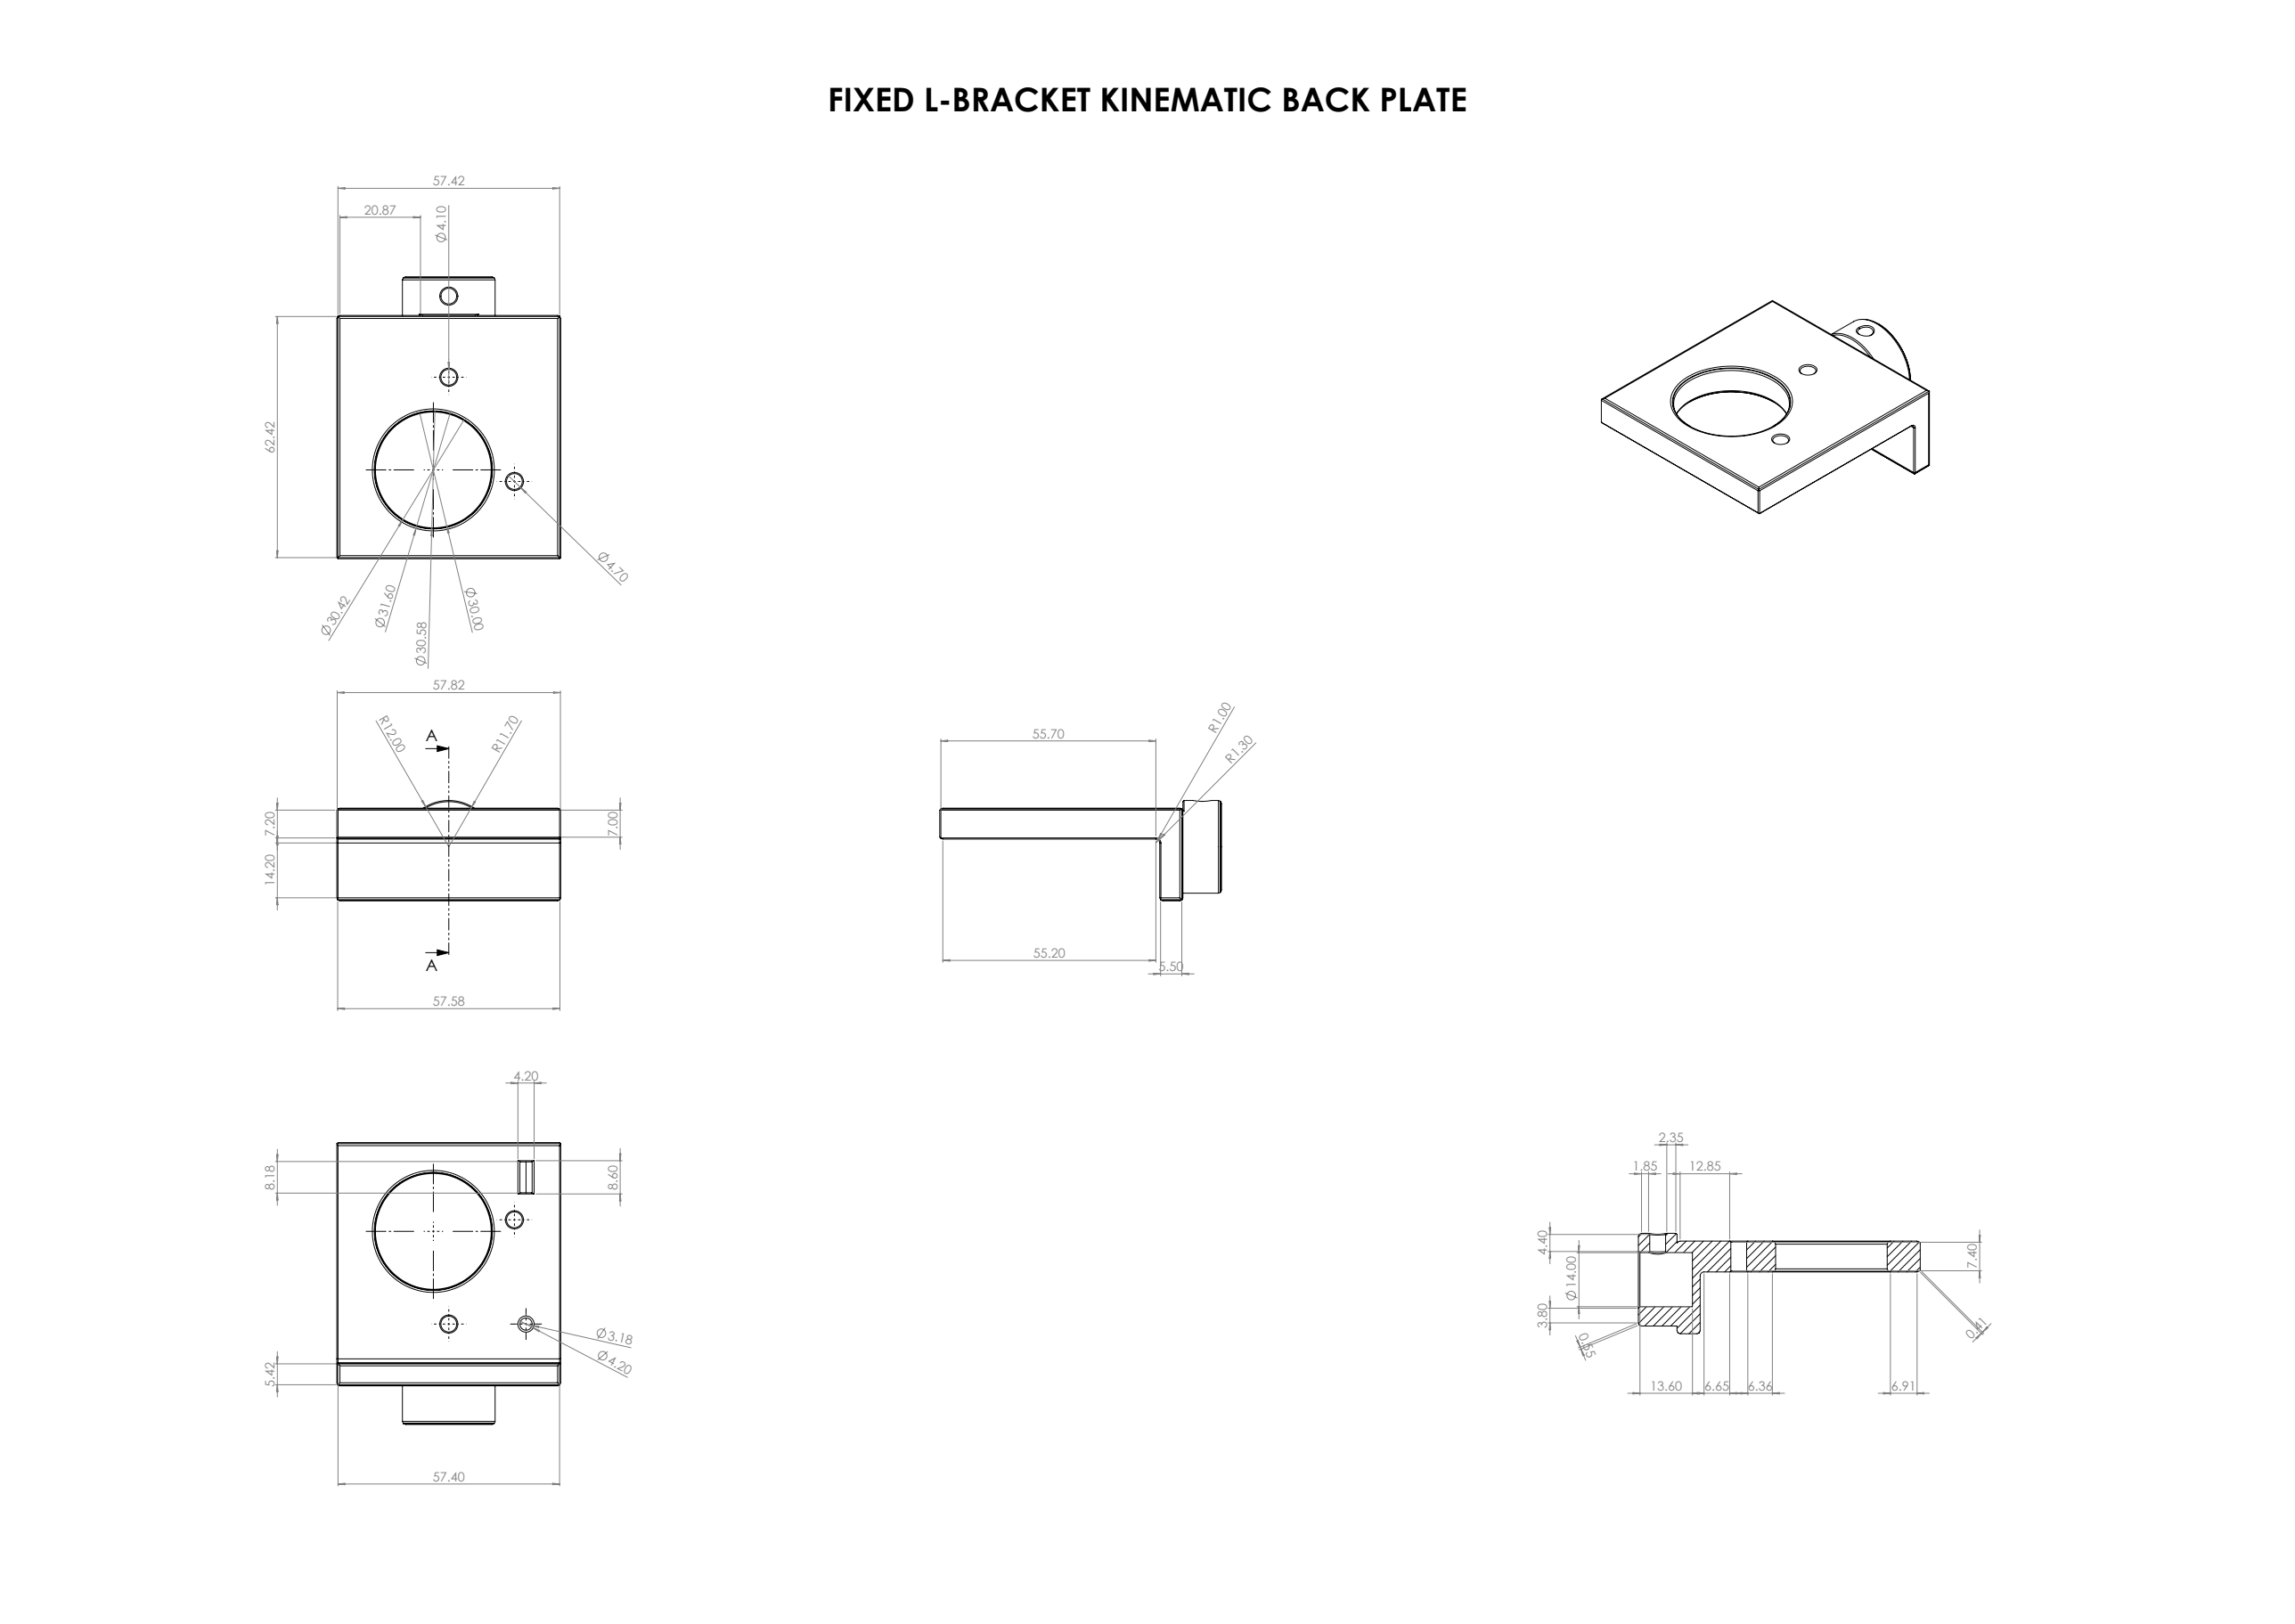
ISO-10303-21;
HEADER;
/* Generated by software containing ST-Developer
 * from STEP Tools, Inc. (www.steptools.com) 
 */

FILE_DESCRIPTION(
/* description */ (''),
/* implementation_level */ '2;1');

FILE_NAME(
/* name */ 
'04_Fixed_L-Bracket_Kinematic_Back_Plate.step',
/* time_stamp */ '2026-10-20T10:06:23-07:00',
/* author */ (''),
/* organization */ (''),
/* preprocessor_version */ 'ST-DEVELOPER v20.2',
/* originating_system */ 'Autodesk Translation Framework v15.15.0.0',
/* authorisation */ '');

FILE_SCHEMA (('AUTOMOTIVE_DESIGN { 1 0 10303 214 3 1 1 }'));
ENDSEC;

DATA;
#10=MECHANICAL_DESIGN_GEOMETRIC_PRESENTATION_REPRESENTATION('',(#468),#38611);
#96=ELLIPSE('',#16996,1.69705627484771,1.2);
#97=ELLIPSE('',#16998,1.69705627484771,1.2);
#130=(
BOUNDED_CURVE()
B_SPLINE_CURVE(2,(#27130,#27131,#27132),.UNSPECIFIED.,.F.,.F.)
B_SPLINE_CURVE_WITH_KNOTS((3,3),(0.245470547469808,0.342025381879347),
 .UNSPECIFIED.)
CURVE()
GEOMETRIC_REPRESENTATION_ITEM()
RATIONAL_B_SPLINE_CURVE((1.,1.,1.))
REPRESENTATION_ITEM('')
);
#131=(
BOUNDED_CURVE()
B_SPLINE_CURVE(2,(#27135,#27136,#27137),.UNSPECIFIED.,.F.,.F.)
B_SPLINE_CURVE_WITH_KNOTS((3,3),(0.165943124807515,0.262497959217054),
 .UNSPECIFIED.)
CURVE()
GEOMETRIC_REPRESENTATION_ITEM()
RATIONAL_B_SPLINE_CURVE((1.,1.,1.))
REPRESENTATION_ITEM('')
);
#440=SHAPE_REPRESENTATION_RELATIONSHIP('SRR','None',#38676,#454);
#454=ADVANCED_BREP_SHAPE_REPRESENTATION('',(#482),#38605);
#468=STYLED_ITEM('',(#38857),#482);
#482=MANIFOLD_SOLID_BREP('Bracket',#16242);
#501=B_SPLINE_SURFACE_WITH_KNOTS('',3,3,((#26897,#26898,#26899,#26900,#26901,
#26902,#26903,#26904,#26905,#26906,#26907,#26908,#26909,#26910,#26911,#26912,
#26913,#26914,#26915,#26916,#26917,#26918,#26919,#26920,#26921,#26922,#26923,
#26924,#26925,#26926),(#26927,#26928,#26929,#26930,#26931,#26932,#26933,
#26934,#26935,#26936,#26937,#26938,#26939,#26940,#26941,#26942,#26943,#26944,
#26945,#26946,#26947,#26948,#26949,#26950,#26951,#26952,#26953,#26954,#26955,
#26956),(#26957,#26958,#26959,#26960,#26961,#26962,#26963,#26964,#26965,
#26966,#26967,#26968,#26969,#26970,#26971,#26972,#26973,#26974,#26975,#26976,
#26977,#26978,#26979,#26980,#26981,#26982,#26983,#26984,#26985,#26986),
(#26987,#26988,#26989,#26990,#26991,#26992,#26993,#26994,#26995,#26996,
#26997,#26998,#26999,#27000,#27001,#27002,#27003,#27004,#27005,#27006,#27007,
#27008,#27009,#27010,#27011,#27012,#27013,#27014,#27015,#27016)),
 .UNSPECIFIED.,.F.,.T.,.F.,(4,4),(4,1,1,1,1,1,1,1,2,2,2,2,1,1,1,1,1,1,1,
2,2,4),(0.,1.),(0.,0.0483649312414982,0.0967298624829964,0.145094793724495,
0.193459724965993,0.241824656207491,0.290189587448989,0.326463285880113,
0.386919449931986,0.464302426118159,0.541687686804892,0.619072947491625,
0.677110750756395,0.735148554021165,0.793186357285935,0.851224160550705,
0.909261963815475,0.967299767080245,0.99631866871263,1.08337537360978,1.16076063429652,
1.23814589498325),.UNSPECIFIED.);
#502=B_SPLINE_SURFACE_WITH_KNOTS('',3,3,((#27146,#27147,#27148,#27149,#27150,
#27151,#27152,#27153,#27154,#27155,#27156,#27157,#27158,#27159,#27160,#27161,
#27162,#27163,#27164,#27165,#27166,#27167,#27168,#27169,#27170,#27171),
(#27172,#27173,#27174,#27175,#27176,#27177,#27178,#27179,#27180,#27181,
#27182,#27183,#27184,#27185,#27186,#27187,#27188,#27189,#27190,#27191,#27192,
#27193,#27194,#27195,#27196,#27197),(#27198,#27199,#27200,#27201,#27202,
#27203,#27204,#27205,#27206,#27207,#27208,#27209,#27210,#27211,#27212,#27213,
#27214,#27215,#27216,#27217,#27218,#27219,#27220,#27221,#27222,#27223),
(#27224,#27225,#27226,#27227,#27228,#27229,#27230,#27231,#27232,#27233,
#27234,#27235,#27236,#27237,#27238,#27239,#27240,#27241,#27242,#27243,#27244,
#27245,#27246,#27247,#27248,#27249)),.UNSPECIFIED.,.F.,.T.,.F.,(4,4),(4,
2,2,2,2,2,1,1,1,1,1,1,1,2,2,1,4),(0.,1.),(0.358934429201528,0.49197868985962,
0.564785636730508,0.596617469546802,0.699442998635822,0.77716819339067,
0.842568141080894,0.907968088771118,0.973368036461342,1.03876798415157,
1.07146795799668,1.10416793184179,1.16956787953201,1.30036777491246,1.39600843428647,
1.50005496459849,1.6041014949105),.UNSPECIFIED.);
#619=B_SPLINE_CURVE_WITH_KNOTS('',3,(#27021,#27022,#27023,#27024,#27025,
#27026,#27027,#27028,#27029,#27030,#27031,#27032,#27033,#27034,#27035,#27036,
#27037,#27038,#27039,#27040,#27041,#27042,#27043,#27044),.UNSPECIFIED.,
 .F.,.F.,(4,1,1,1,1,1,1,1,2,2,2,2,1,1,1,1,1,4),(0.,0.0483649312414982,0.0967298624829964,
0.145094793724495,0.193459724965993,0.241824656207491,0.290189587448989,
0.326463285880113,0.386919449931986,0.464302426118159,0.541687686804892,
0.619072947491625,0.677110750756395,0.735148554021165,0.793186357285935,
0.851224160550705,0.909261963815475,0.928609421237438),.UNSPECIFIED.);
#620=B_SPLINE_CURVE_WITH_KNOTS('',3,(#27045,#27046,#27047,#27048,#27049,
#27050,#27051,#27052,#27053,#27054),.UNSPECIFIED.,.F.,.F.,(4,1,1,2,2,4),
(0.928609421237438,0.967299767080245,0.99631866871263,1.08337537360978,
1.16076063429652,1.23814589498325),.UNSPECIFIED.);
#621=B_SPLINE_CURVE_WITH_KNOTS('',3,(#27055,#27056,#27057,#27058,#27059,
#27060,#27061,#27062,#27063,#27064,#27065,#27066,#27067,#27068,#27069,#27070,
#27071,#27072,#27073,#27074,#27075,#27076,#27077,#27078,#27079,#27080,#27081,
#27082,#27083,#27084),.UNSPECIFIED.,.T.,.F.,(4,2,2,1,1,1,1,1,1,1,2,2,2,
2,1,1,1,1,1,1,1,4),(-1.23814589498325,-1.16076063429652,-1.08337537360978,
-0.99631866871263,-0.967299767080245,-0.909261963815475,-0.851224160550705,
-0.793186357285935,-0.735148554021165,-0.677110750756395,-0.619072947491625,
-0.541687686804892,-0.464302426118159,-0.386919449931986,-0.326463285880113,
-0.290189587448989,-0.241824656207491,-0.193459724965993,-0.145094793724495,
-0.0967298624829964,-0.0483649312414982,0.),.UNSPECIFIED.);
#622=B_SPLINE_CURVE_WITH_KNOTS('',3,(#27097,#27098,#27099,#27100,#27101,
#27102,#27103,#27104,#27105,#27106,#27107,#27108,#27109,#27110,#27111,#27112),
 .UNSPECIFIED.,.F.,.F.,(4,2,2,2,2,2,1,1,4),(0.358934429201528,0.49197868985962,
0.564785636730508,0.596617469546802,0.699442998635822,0.77716819339067,
0.842568141080894,0.907968088771118,0.932576705821461),.UNSPECIFIED.);
#623=B_SPLINE_CURVE_WITH_KNOTS('',3,(#27113,#27114,#27115,#27116,#27117,
#27118,#27119,#27120,#27121,#27122,#27123,#27124,#27125,#27126),
 .UNSPECIFIED.,.F.,.F.,(4,1,1,1,1,1,2,2,1,4),(0.932576705821461,0.973368036461342,
1.03876798415157,1.07146795799668,1.10416793184179,1.16956787953201,1.30036777491246,
1.39600843428647,1.50005496459849,1.6041014949105),.UNSPECIFIED.);
#624=B_SPLINE_CURVE_WITH_KNOTS('',3,(#27253,#27254,#27255,#27256,#27257,
#27258,#27259,#27260,#27261,#27262),.UNSPECIFIED.,.F.,.F.,(4,1,2,2,1,4),
(-1.6041014949105,-1.50005496459849,-1.39600843428647,-1.30036777491246,
-1.16956787953201,-1.14109494863627),.UNSPECIFIED.);
#625=B_SPLINE_CURVE_WITH_KNOTS('',3,(#27264,#27265,#27266,#27267,#27268,
#27269,#27270,#27271,#27272,#27273,#27274,#27275),.UNSPECIFIED.,.F.,.F.,
(4,1,1,1,1,1,1,2,4),(-1.14109494863627,-1.10416793184179,-1.07146795799668,
-1.03876798415157,-0.973368036461342,-0.907968088771118,-0.842568141080894,
-0.77716819339067,-0.72405846300665),.UNSPECIFIED.);
#626=B_SPLINE_CURVE_WITH_KNOTS('',3,(#27276,#27277,#27278,#27279,#27280,
#27281,#27282,#27283,#27284,#27285,#27286,#27287),.UNSPECIFIED.,.F.,.F.,
(4,2,2,2,2,4),(-0.72405846300665,-0.699442998635822,-0.596617469546802,
-0.564785636730508,-0.49197868985962,-0.358934429201528),.UNSPECIFIED.);
#942=CYLINDRICAL_SURFACE('',#16994,1.2);
#943=CYLINDRICAL_SURFACE('',#16999,0.204999999999999);
#944=CYLINDRICAL_SURFACE('',#17006,0.7);
#945=CYLINDRICAL_SURFACE('',#17051,0.205);
#946=CYLINDRICAL_SURFACE('',#17055,0.205);
#947=CYLINDRICAL_SURFACE('',#17081,1.5);
#948=CYLINDRICAL_SURFACE('',#17097,0.1);
#1188=FACE_BOUND('',#3107,.T.);
#1189=FACE_BOUND('',#3114,.T.);
#1190=FACE_BOUND('',#3117,.T.);
#1191=FACE_BOUND('',#3146,.T.);
#1192=FACE_BOUND('',#3147,.T.);
#1193=FACE_BOUND('',#3148,.T.);
#1194=FACE_BOUND('',#3149,.T.);
#1195=FACE_BOUND('',#3150,.T.);
#1196=FACE_BOUND('',#3165,.T.);
#1197=FACE_BOUND('',#3166,.T.);
#1198=FACE_BOUND('',#3167,.T.);
#1410=CIRCLE('',#16992,1.2);
#1411=CIRCLE('',#16993,1.2);
#1412=CIRCLE('',#16995,1.2);
#1413=CIRCLE('',#16997,1.2);
#1414=CIRCLE('',#17001,1.17);
#1415=CIRCLE('',#17003,1.1787867965644);
#1416=CIRCLE('',#17005,1.1712132034356);
#1417=CIRCLE('',#17007,0.7);
#1418=CIRCLE('',#17008,0.7);
#1419=CIRCLE('',#17010,1.12);
#1420=CIRCLE('',#17012,0.74);
#1421=CIRCLE('',#17031,0.13);
#1422=CIRCLE('',#17042,0.21);
#1423=CIRCLE('',#17043,0.234999999999999);
#1424=CIRCLE('',#17044,1.58);
#1425=CIRCLE('',#17045,0.235);
#1426=CIRCLE('',#17047,0.158786796564404);
#1427=CIRCLE('',#17050,0.205);
#1428=CIRCLE('',#17052,0.205);
#1429=CIRCLE('',#17054,0.205);
#1430=CIRCLE('',#17056,0.205);
#1431=CIRCLE('',#17058,0.1);
#1432=CIRCLE('',#17061,0.1);
#1433=CIRCLE('',#17062,0.13);
#1434=CIRCLE('',#17065,1.5287867965644);
#1435=CIRCLE('',#17067,1.5212132034356);
#1436=CIRCLE('',#17069,0.235);
#1437=CIRCLE('',#17071,0.234999999999999);
#1438=CIRCLE('',#17072,1.58);
#1439=CIRCLE('',#17080,1.5);
#1440=CIRCLE('',#17082,1.5);
#1441=CIRCLE('',#17084,1.5287867965644);
#1442=CIRCLE('',#17086,1.5212132034356);
#1746=CONICAL_SURFACE('',#17000,1.185,0.785398163397445);
#1747=CONICAL_SURFACE('',#17002,1.1893933982822,0.392699081698718);
#1748=CONICAL_SURFACE('',#17004,1.175,0.785398163397451);
#1749=CONICAL_SURFACE('',#17009,1.1456066017178,1.17809724509618);
#1750=CONICAL_SURFACE('',#17046,0.184393398282202,1.17809724509617);
#1751=CONICAL_SURFACE('',#17048,0.115,0.785398163397448);
#1752=CONICAL_SURFACE('',#17049,0.22,0.785398163397453);
#1753=CONICAL_SURFACE('',#17053,0.22,0.785398163397438);
#1754=CONICAL_SURFACE('',#17057,0.115,0.785398163397456);
#1755=CONICAL_SURFACE('',#17060,0.115,0.785398163397456);
#1756=CONICAL_SURFACE('',#17064,1.5543933982822,1.17809724509617);
#1757=CONICAL_SURFACE('',#17066,1.525,0.785398163397449);
#1758=CONICAL_SURFACE('',#17068,0.22,0.785398163397452);
#1759=CONICAL_SURFACE('',#17073,0.22,0.785398163397437);
#1760=CONICAL_SURFACE('',#17079,1.5106066017178,0.392699081698724);
#1761=CONICAL_SURFACE('',#17083,1.5543933982822,1.17809724509617);
#1762=CONICAL_SURFACE('',#17085,1.525,0.785398163397448);
#1763=CONICAL_SURFACE('',#17087,1.5106066017178,0.392699081698721);
#1764=CONICAL_SURFACE('',#17090,0.72,0.785398163397448);
#2151=FACE_OUTER_BOUND('',#3097,.T.);
#2152=FACE_OUTER_BOUND('',#3098,.T.);
#2153=FACE_OUTER_BOUND('',#3099,.T.);
#2154=FACE_OUTER_BOUND('',#3100,.T.);
#2155=FACE_OUTER_BOUND('',#3101,.T.);
#2156=FACE_OUTER_BOUND('',#3102,.T.);
#2157=FACE_OUTER_BOUND('',#3103,.T.);
#2158=FACE_OUTER_BOUND('',#3104,.T.);
#2159=FACE_OUTER_BOUND('',#3105,.T.);
#2160=FACE_OUTER_BOUND('',#3106,.T.);
#2161=FACE_OUTER_BOUND('',#3108,.T.);
#2162=FACE_OUTER_BOUND('',#3109,.T.);
#2163=FACE_OUTER_BOUND('',#3110,.T.);
#2164=FACE_OUTER_BOUND('',#3111,.T.);
#2165=FACE_OUTER_BOUND('',#3112,.T.);
#2166=FACE_OUTER_BOUND('',#3113,.T.);
#2167=FACE_OUTER_BOUND('',#3115,.T.);
#2168=FACE_OUTER_BOUND('',#3116,.T.);
#2169=FACE_OUTER_BOUND('',#3118,.T.);
#2170=FACE_OUTER_BOUND('',#3119,.T.);
#2171=FACE_OUTER_BOUND('',#3120,.T.);
#2172=FACE_OUTER_BOUND('',#3121,.T.);
#2173=FACE_OUTER_BOUND('',#3122,.T.);
#2174=FACE_OUTER_BOUND('',#3123,.T.);
#2175=FACE_OUTER_BOUND('',#3124,.T.);
#2176=FACE_OUTER_BOUND('',#3125,.T.);
#2177=FACE_OUTER_BOUND('',#3126,.T.);
#2178=FACE_OUTER_BOUND('',#3127,.T.);
#2179=FACE_OUTER_BOUND('',#3128,.T.);
#2180=FACE_OUTER_BOUND('',#3129,.T.);
#2181=FACE_OUTER_BOUND('',#3130,.T.);
#2182=FACE_OUTER_BOUND('',#3131,.T.);
#2183=FACE_OUTER_BOUND('',#3132,.T.);
#2184=FACE_OUTER_BOUND('',#3133,.T.);
#2185=FACE_OUTER_BOUND('',#3134,.T.);
#2186=FACE_OUTER_BOUND('',#3135,.T.);
#2187=FACE_OUTER_BOUND('',#3136,.T.);
#2188=FACE_OUTER_BOUND('',#3137,.T.);
#2189=FACE_OUTER_BOUND('',#3138,.T.);
#2190=FACE_OUTER_BOUND('',#3139,.T.);
#2191=FACE_OUTER_BOUND('',#3140,.T.);
#2192=FACE_OUTER_BOUND('',#3141,.T.);
#2193=FACE_OUTER_BOUND('',#3142,.T.);
#2194=FACE_OUTER_BOUND('',#3143,.T.);
#2195=FACE_OUTER_BOUND('',#3144,.T.);
#2196=FACE_OUTER_BOUND('',#3145,.T.);
#2197=FACE_OUTER_BOUND('',#3151,.T.);
#2198=FACE_OUTER_BOUND('',#3152,.T.);
#2199=FACE_OUTER_BOUND('',#3153,.T.);
#2200=FACE_OUTER_BOUND('',#3154,.T.);
#2201=FACE_OUTER_BOUND('',#3155,.T.);
#2202=FACE_OUTER_BOUND('',#3156,.T.);
#2203=FACE_OUTER_BOUND('',#3157,.T.);
#2204=FACE_OUTER_BOUND('',#3158,.T.);
#2205=FACE_OUTER_BOUND('',#3159,.T.);
#2206=FACE_OUTER_BOUND('',#3160,.T.);
#2207=FACE_OUTER_BOUND('',#3161,.T.);
#2208=FACE_OUTER_BOUND('',#3162,.T.);
#2209=FACE_OUTER_BOUND('',#3163,.T.);
#2210=FACE_OUTER_BOUND('',#3164,.T.);
#2211=FACE_OUTER_BOUND('',#3168,.T.);
#2212=FACE_OUTER_BOUND('',#3169,.T.);
#2213=FACE_OUTER_BOUND('',#3170,.T.);
#2214=FACE_OUTER_BOUND('',#3171,.T.);
#2215=FACE_OUTER_BOUND('',#3172,.T.);
#2216=FACE_OUTER_BOUND('',#3173,.T.);
#2217=FACE_OUTER_BOUND('',#3174,.T.);
#2218=FACE_OUTER_BOUND('',#3175,.T.);
#2219=FACE_OUTER_BOUND('',#3176,.T.);
#2220=FACE_OUTER_BOUND('',#3177,.T.);
#2221=FACE_OUTER_BOUND('',#3178,.T.);
#2222=FACE_OUTER_BOUND('',#3179,.T.);
#2223=FACE_OUTER_BOUND('',#3180,.T.);
#2224=FACE_OUTER_BOUND('',#3181,.T.);
#2225=FACE_OUTER_BOUND('',#3182,.T.);
#2226=FACE_OUTER_BOUND('',#3183,.T.);
#2227=FACE_OUTER_BOUND('',#3184,.T.);
#2228=FACE_OUTER_BOUND('',#3185,.T.);
#2229=FACE_OUTER_BOUND('',#3186,.T.);
#2230=FACE_OUTER_BOUND('',#3187,.T.);
#2231=FACE_OUTER_BOUND('',#3188,.T.);
#3097=EDGE_LOOP('',(#11825,#11826,#11827,#11828,#11829,#11830));
#3098=EDGE_LOOP('',(#11831,#11832,#11833,#11834,#11835));
#3099=EDGE_LOOP('',(#11836,#11837,#11838,#11839,#11840));
#3100=EDGE_LOOP('',(#11841,#11842,#11843,#11844));
#3101=EDGE_LOOP('',(#11845,#11846,#11847,#11848));
#3102=EDGE_LOOP('',(#11849,#11850,#11851,#11852));
#3103=EDGE_LOOP('',(#11853,#11854,#11855,#11856));
#3104=EDGE_LOOP('',(#11857,#11858,#11859,#11860,#11861,#11862,#11863));
#3105=EDGE_LOOP('',(#11864,#11865,#11866,#11867,#11868));
#3106=EDGE_LOOP('',(#11869,#11870,#11871,#11872,#11873,#11874,#11875,#11876));
#3107=EDGE_LOOP('',(#11877));
#3108=EDGE_LOOP('',(#11878,#11879,#11880,#11881,#11882,#11883));
#3109=EDGE_LOOP('',(#11884,#11885,#11886,#11887));
#3110=EDGE_LOOP('',(#11888,#11889,#11890,#11891));
#3111=EDGE_LOOP('',(#11892,#11893,#11894,#11895));
#3112=EDGE_LOOP('',(#11896,#11897,#11898,#11899,#11900,#11901,#11902));
#3113=EDGE_LOOP('',(#11903,#11904,#11905,#11906));
#3114=EDGE_LOOP('',(#11907,#11908,#11909));
#3115=EDGE_LOOP('',(#11910,#11911,#11912,#11913));
#3116=EDGE_LOOP('',(#11914));
#3117=EDGE_LOOP('',(#11915));
#3118=EDGE_LOOP('',(#11916,#11917,#11918,#11919));
#3119=EDGE_LOOP('',(#11920,#11921,#11922,#11923));
#3120=EDGE_LOOP('',(#11924,#11925,#11926,#11927));
#3121=EDGE_LOOP('',(#11928,#11929,#11930,#11931));
#3122=EDGE_LOOP('',(#11932,#11933,#11934,#11935,#11936));
#3123=EDGE_LOOP('',(#11937,#11938,#11939,#11940));
#3124=EDGE_LOOP('',(#11941,#11942,#11943,#11944,#11945,#11946));
#3125=EDGE_LOOP('',(#11947,#11948,#11949,#11950,#11951,#11952));
#3126=EDGE_LOOP('',(#11953,#11954,#11955,#11956,#11957,#11958));
#3127=EDGE_LOOP('',(#11959,#11960,#11961,#11962));
#3128=EDGE_LOOP('',(#11963,#11964,#11965,#11966));
#3129=EDGE_LOOP('',(#11967,#11968,#11969,#11970,#11971,#11972,#11973));
#3130=EDGE_LOOP('',(#11974,#11975,#11976,#11977,#11978,#11979));
#3131=EDGE_LOOP('',(#11980,#11981,#11982,#11983,#11984));
#3132=EDGE_LOOP('',(#11985,#11986,#11987,#11988));
#3133=EDGE_LOOP('',(#11989,#11990,#11991,#11992,#11993));
#3134=EDGE_LOOP('',(#11994,#11995,#11996,#11997,#11998,#11999,#12000));
#3135=EDGE_LOOP('',(#12001,#12002,#12003,#12004,#12005,#12006,#12007));
#3136=EDGE_LOOP('',(#12008,#12009,#12010,#12011,#12012));
#3137=EDGE_LOOP('',(#12013,#12014,#12015,#12016,#12017,#12018));
#3138=EDGE_LOOP('',(#12019,#12020,#12021,#12022,#12023,#12024));
#3139=EDGE_LOOP('',(#12025,#12026,#12027,#12028));
#3140=EDGE_LOOP('',(#12029,#12030,#12031,#12032));
#3141=EDGE_LOOP('',(#12033,#12034,#12035,#12036,#12037,#12038));
#3142=EDGE_LOOP('',(#12039,#12040,#12041,#12042,#12043,#12044));
#3143=EDGE_LOOP('',(#12045,#12046,#12047));
#3144=EDGE_LOOP('',(#12048,#12049,#12050,#12051,#12052,#12053));
#3145=EDGE_LOOP('',(#12054,#12055,#12056,#12057));
#3146=EDGE_LOOP('',(#12058));
#3147=EDGE_LOOP('',(#12059));
#3148=EDGE_LOOP('',(#12060));
#3149=EDGE_LOOP('',(#12061));
#3150=EDGE_LOOP('',(#12062,#12063,#12064,#12065));
#3151=EDGE_LOOP('',(#12066,#12067,#12068,#12069));
#3152=EDGE_LOOP('',(#12070,#12071,#12072));
#3153=EDGE_LOOP('',(#12073,#12074,#12075,#12076));
#3154=EDGE_LOOP('',(#12077,#12078,#12079,#12080));
#3155=EDGE_LOOP('',(#12081,#12082,#12083,#12084));
#3156=EDGE_LOOP('',(#12085,#12086,#12087,#12088));
#3157=EDGE_LOOP('',(#12089,#12090,#12091,#12092));
#3158=EDGE_LOOP('',(#12093,#12094,#12095,#12096));
#3159=EDGE_LOOP('',(#12097,#12098,#12099,#12100));
#3160=EDGE_LOOP('',(#12101,#12102,#12103,#12104,#12105,#12106,#12107));
#3161=EDGE_LOOP('',(#12108,#12109,#12110,#12111));
#3162=EDGE_LOOP('',(#12112,#12113,#12114,#12115));
#3163=EDGE_LOOP('',(#12116,#12117,#12118,#12119));
#3164=EDGE_LOOP('',(#12120,#12121,#12122,#12123));
#3165=EDGE_LOOP('',(#12124));
#3166=EDGE_LOOP('',(#12125));
#3167=EDGE_LOOP('',(#12126));
#3168=EDGE_LOOP('',(#12127,#12128,#12129,#12130));
#3169=EDGE_LOOP('',(#12131,#12132,#12133,#12134));
#3170=EDGE_LOOP('',(#12135,#12136,#12137,#12138));
#3171=EDGE_LOOP('',(#12139,#12140,#12141,#12142));
#3172=EDGE_LOOP('',(#12143,#12144,#12145,#12146));
#3173=EDGE_LOOP('',(#12147,#12148,#12149,#12150,#12151,#12152,#12153,#12154,
#12155,#12156,#12157,#12158,#12159,#12160));
#3174=EDGE_LOOP('',(#12161,#12162,#12163,#12164));
#3175=EDGE_LOOP('',(#12165,#12166,#12167,#12168));
#3176=EDGE_LOOP('',(#12169,#12170,#12171,#12172));
#3177=EDGE_LOOP('',(#12173,#12174,#12175,#12176));
#3178=EDGE_LOOP('',(#12177,#12178,#12179,#12180));
#3179=EDGE_LOOP('',(#12181,#12182,#12183,#12184,#12185,#12186));
#3180=EDGE_LOOP('',(#12187,#12188,#12189));
#3181=EDGE_LOOP('',(#12190,#12191,#12192,#12193));
#3182=EDGE_LOOP('',(#12194));
#3183=EDGE_LOOP('',(#12195,#12196));
#3184=EDGE_LOOP('',(#12197,#12198,#12199,#12200,#12201,#12202));
#3185=EDGE_LOOP('',(#12203,#12204,#12205,#12206,#12207,#12208));
#3186=EDGE_LOOP('',(#12209,#12210,#12211,#12212,#12213,#12214));
#3187=EDGE_LOOP('',(#12215,#12216,#12217,#12218));
#3188=EDGE_LOOP('',(#12219,#12220,#12221,#12222));
#4211=LINE('',#26838,#5435);
#4212=LINE('',#26840,#5436);
#4213=LINE('',#26842,#5437);
#4214=LINE('',#26844,#5438);
#4215=LINE('',#26846,#5439);
#4216=LINE('',#26847,#5440);
#4217=LINE('',#26850,#5441);
#4218=LINE('',#26852,#5442);
#4219=LINE('',#26854,#5443);
#4220=LINE('',#26855,#5444);
#4221=LINE('',#26858,#5445);
#4222=LINE('',#26860,#5446);
#4223=LINE('',#26861,#5447);
#4224=LINE('',#26864,#5448);
#4225=LINE('',#26866,#5449);
#4226=LINE('',#26867,#5450);
#4227=LINE('',#26871,#5451);
#4228=LINE('',#26873,#5452);
#4229=LINE('',#26875,#5453);
#4230=LINE('',#26876,#5454);
#4231=LINE('',#26879,#5455);
#4232=LINE('',#26881,#5456);
#4233=LINE('',#26882,#5457);
#4234=LINE('',#26885,#5458);
#4235=LINE('',#26887,#5459);
#4236=LINE('',#26888,#5460);
#4237=LINE('',#26891,#5461);
#4238=LINE('',#26896,#5462);
#4239=LINE('',#27019,#5463);
#4240=LINE('',#27088,#5464);
#4241=LINE('',#27127,#5465);
#4242=LINE('',#27141,#5466);
#4243=LINE('',#27145,#5467);
#4244=LINE('',#27251,#5468);
#4245=LINE('',#27292,#5469);
#4246=LINE('',#27296,#5470);
#4247=LINE('',#27304,#5471);
#4248=LINE('',#27306,#5472);
#4249=LINE('',#27308,#5473);
#4250=LINE('',#27309,#5474);
#4251=LINE('',#27313,#5475);
#4252=LINE('',#27314,#5476);
#4253=LINE('',#27315,#5477);
#4254=LINE('',#27317,#5478);
#4255=LINE('',#27318,#5479);
#4256=LINE('',#27320,#5480);
#4257=LINE('',#27321,#5481);
#4258=LINE('',#27324,#5482);
#4259=LINE('',#27326,#5483);
#4260=LINE('',#27327,#5484);
#4261=LINE('',#27332,#5485);
#4262=LINE('',#27334,#5486);
#4263=LINE('',#27336,#5487);
#4264=LINE('',#27338,#5488);
#4265=LINE('',#27340,#5489);
#4266=LINE('',#27341,#5490);
#4267=LINE('',#27344,#5491);
#4268=LINE('',#27346,#5492);
#4269=LINE('',#27348,#5493);
#4270=LINE('',#27350,#5494);
#4271=LINE('',#27351,#5495);
#4272=LINE('',#27354,#5496);
#4273=LINE('',#27356,#5497);
#4274=LINE('',#27358,#5498);
#4275=LINE('',#27359,#5499);
#4276=LINE('',#27362,#5500);
#4277=LINE('',#27363,#5501);
#4278=LINE('',#27366,#5502);
#4279=LINE('',#27368,#5503);
#4280=LINE('',#27369,#5504);
#4281=LINE('',#27371,#5505);
#4282=LINE('',#27373,#5506);
#4283=LINE('',#27375,#5507);
#4284=LINE('',#27377,#5508);
#4285=LINE('',#27378,#5509);
#4286=LINE('',#27380,#5510);
#4287=LINE('',#27382,#5511);
#4288=LINE('',#27383,#5512);
#4289=LINE('',#27385,#5513);
#4290=LINE('',#27389,#5514);
#4291=LINE('',#27391,#5515);
#4292=LINE('',#27392,#5516);
#4293=LINE('',#27393,#5517);
#4294=LINE('',#27396,#5518);
#4295=LINE('',#27397,#5519);
#4296=LINE('',#27400,#5520);
#4297=LINE('',#27402,#5521);
#4298=LINE('',#27404,#5522);
#4299=LINE('',#27406,#5523);
#4300=LINE('',#27408,#5524);
#4301=LINE('',#27409,#5525);
#4302=LINE('',#27412,#5526);
#4303=LINE('',#27416,#5527);
#4304=LINE('',#27417,#5528);
#4305=LINE('',#27420,#5529);
#4306=LINE('',#27421,#5530);
#4307=LINE('',#27423,#5531);
#4308=LINE('',#27424,#5532);
#4309=LINE('',#27427,#5533);
#4310=LINE('',#27429,#5534);
#4311=LINE('',#27430,#5535);
#4312=LINE('',#27434,#5536);
#4313=LINE('',#27436,#5537);
#4314=LINE('',#27438,#5538);
#4315=LINE('',#27439,#5539);
#4316=LINE('',#27443,#5540);
#4317=LINE('',#27445,#5541);
#4318=LINE('',#27447,#5542);
#4319=LINE('',#27448,#5543);
#4320=LINE('',#27452,#5544);
#4321=LINE('',#27453,#5545);
#4322=LINE('',#27454,#5546);
#4323=LINE('',#27455,#5547);
#4324=LINE('',#27457,#5548);
#4325=LINE('',#27459,#5549);
#4326=LINE('',#27461,#5550);
#4327=LINE('',#27462,#5551);
#4328=LINE('',#27465,#5552);
#4329=LINE('',#27466,#5553);
#4330=LINE('',#27469,#5554);
#4331=LINE('',#27470,#5555);
#4332=LINE('',#27472,#5556);
#4333=LINE('',#27473,#5557);
#4334=LINE('',#27484,#5558);
#4335=LINE('',#27488,#5559);
#4336=LINE('',#27491,#5560);
#4337=LINE('',#27495,#5561);
#4338=LINE('',#27499,#5562);
#4339=LINE('',#27503,#5563);
#4340=LINE('',#27515,#5564);
#4341=LINE('',#27518,#5565);
#4342=LINE('',#27523,#5566);
#4343=LINE('',#27527,#5567);
#4344=LINE('',#27529,#5568);
#4345=LINE('',#27531,#5569);
#4346=LINE('',#27532,#5570);
#4347=LINE('',#27538,#5571);
#4348=LINE('',#27540,#5572);
#4349=LINE('',#27541,#5573);
#4350=LINE('',#27542,#5574);
#4351=LINE('',#27544,#5575);
#4352=LINE('',#27545,#5576);
#4353=LINE('',#27546,#5577);
#4354=LINE('',#27550,#5578);
#4355=LINE('',#27551,#5579);
#4356=LINE('',#27554,#5580);
#4357=LINE('',#27559,#5581);
#4358=LINE('',#27563,#5582);
#4359=LINE('',#27566,#5583);
#4360=LINE('',#27569,#5584);
#4361=LINE('',#27571,#5585);
#4362=LINE('',#27574,#5586);
#4363=LINE('',#27578,#5587);
#4364=LINE('',#27582,#5588);
#5435=VECTOR('',#19526,1.);
#5436=VECTOR('',#19527,1.);
#5437=VECTOR('',#19528,1.);
#5438=VECTOR('',#19529,1.);
#5439=VECTOR('',#19530,1.);
#5440=VECTOR('',#19531,1.);
#5441=VECTOR('',#19534,1.);
#5442=VECTOR('',#19535,1.);
#5443=VECTOR('',#19536,1.);
#5444=VECTOR('',#19537,1.);
#5445=VECTOR('',#19540,1.);
#5446=VECTOR('',#19541,1.);
#5447=VECTOR('',#19542,1.);
#5448=VECTOR('',#19545,1.);
#5449=VECTOR('',#19546,1.);
#5450=VECTOR('',#19547,1.);
#5451=VECTOR('',#19550,1.);
#5452=VECTOR('',#19551,1.);
#5453=VECTOR('',#19552,1.);
#5454=VECTOR('',#19553,1.);
#5455=VECTOR('',#19556,1.);
#5456=VECTOR('',#19557,1.);
#5457=VECTOR('',#19558,1.);
#5458=VECTOR('',#19561,1.);
#5459=VECTOR('',#19562,1.);
#5460=VECTOR('',#19563,1.);
#5461=VECTOR('',#19566,1.);
#5462=VECTOR('',#19571,1.);
#5463=VECTOR('',#19572,1.);
#5464=VECTOR('',#19577,1.2);
#5465=VECTOR('',#19586,0.204999999999999);
#5466=VECTOR('',#19595,1.1893933982822);
#5467=VECTOR('',#19600,1.175);
#5468=VECTOR('',#19601,1.);
#5469=VECTOR('',#19606,0.7);
#5470=VECTOR('',#19611,1.1456066017178);
#5471=VECTOR('',#19620,1.);
#5472=VECTOR('',#19621,1.);
#5473=VECTOR('',#19622,1.);
#5474=VECTOR('',#19623,1.);
#5475=VECTOR('',#19626,1.);
#5476=VECTOR('',#19627,1.);
#5477=VECTOR('',#19628,1.);
#5478=VECTOR('',#19631,1.);
#5479=VECTOR('',#19632,1.);
#5480=VECTOR('',#19635,1.);
#5481=VECTOR('',#19636,1.);
#5482=VECTOR('',#19639,1.);
#5483=VECTOR('',#19640,1.);
#5484=VECTOR('',#19641,1.);
#5485=VECTOR('',#19646,1.);
#5486=VECTOR('',#19647,1.);
#5487=VECTOR('',#19648,1.);
#5488=VECTOR('',#19649,1.);
#5489=VECTOR('',#19650,1.);
#5490=VECTOR('',#19651,1.);
#5491=VECTOR('',#19654,1.);
#5492=VECTOR('',#19655,1.);
#5493=VECTOR('',#19656,1.);
#5494=VECTOR('',#19657,1.);
#5495=VECTOR('',#19658,1.);
#5496=VECTOR('',#19661,1.);
#5497=VECTOR('',#19662,1.);
#5498=VECTOR('',#19663,1.);
#5499=VECTOR('',#19664,1.);
#5500=VECTOR('',#19667,1.);
#5501=VECTOR('',#19668,1.);
#5502=VECTOR('',#19671,1.);
#5503=VECTOR('',#19672,1.);
#5504=VECTOR('',#19673,1.);
#5505=VECTOR('',#19676,1.);
#5506=VECTOR('',#19677,1.);
#5507=VECTOR('',#19678,1.);
#5508=VECTOR('',#19679,1.);
#5509=VECTOR('',#19680,1.);
#5510=VECTOR('',#19683,1.);
#5511=VECTOR('',#19684,1.);
#5512=VECTOR('',#19685,1.);
#5513=VECTOR('',#19688,1.);
#5514=VECTOR('',#19691,1.);
#5515=VECTOR('',#19692,1.);
#5516=VECTOR('',#19693,1.);
#5517=VECTOR('',#19694,1.);
#5518=VECTOR('',#19697,1.);
#5519=VECTOR('',#19698,1.);
#5520=VECTOR('',#19701,1.);
#5521=VECTOR('',#19702,1.);
#5522=VECTOR('',#19703,1.);
#5523=VECTOR('',#19704,1.);
#5524=VECTOR('',#19705,1.);
#5525=VECTOR('',#19706,1.);
#5526=VECTOR('',#19709,1.);
#5527=VECTOR('',#19712,1.);
#5528=VECTOR('',#19713,1.);
#5529=VECTOR('',#19716,1.);
#5530=VECTOR('',#19717,1.);
#5531=VECTOR('',#19720,1.);
#5532=VECTOR('',#19721,1.);
#5533=VECTOR('',#19724,1.);
#5534=VECTOR('',#19725,1.);
#5535=VECTOR('',#19726,1.);
#5536=VECTOR('',#19729,1.);
#5537=VECTOR('',#19730,1.);
#5538=VECTOR('',#19731,1.);
#5539=VECTOR('',#19732,1.);
#5540=VECTOR('',#19735,1.);
#5541=VECTOR('',#19736,1.);
#5542=VECTOR('',#19737,1.);
#5543=VECTOR('',#19738,1.);
#5544=VECTOR('',#19741,1.);
#5545=VECTOR('',#19742,1.);
#5546=VECTOR('',#19743,1.);
#5547=VECTOR('',#19744,1.);
#5548=VECTOR('',#19747,1.);
#5549=VECTOR('',#19748,1.);
#5550=VECTOR('',#19749,1.);
#5551=VECTOR('',#19750,1.);
#5552=VECTOR('',#19753,1.);
#5553=VECTOR('',#19754,1.);
#5554=VECTOR('',#19757,1.);
#5555=VECTOR('',#19758,1.);
#5556=VECTOR('',#19761,1.);
#5557=VECTOR('',#19762,1.);
#5558=VECTOR('',#19773,0.184393398282202);
#5559=VECTOR('',#19778,0.115);
#5560=VECTOR('',#19781,0.22);
#5561=VECTOR('',#19786,0.205);
#5562=VECTOR('',#19791,0.22);
#5563=VECTOR('',#19796,0.205);
#5564=VECTOR('',#19817,1.5543933982822);
#5565=VECTOR('',#19820,1.525);
#5566=VECTOR('',#19827,0.22);
#5567=VECTOR('',#19830,1.);
#5568=VECTOR('',#19831,1.);
#5569=VECTOR('',#19832,1.);
#5570=VECTOR('',#19833,1.);
#5571=VECTOR('',#19840,0.22);
#5572=VECTOR('',#19843,1.);
#5573=VECTOR('',#19844,1.);
#5574=VECTOR('',#19845,1.);
#5575=VECTOR('',#19848,1.);
#5576=VECTOR('',#19849,1.);
#5577=VECTOR('',#19850,1.);
#5578=VECTOR('',#19857,1.);
#5579=VECTOR('',#19858,1.);
#5580=VECTOR('',#19861,1.5106066017178);
#5581=VECTOR('',#19868,1.5);
#5582=VECTOR('',#19873,1.5543933982822);
#5583=VECTOR('',#19876,1.525);
#5584=VECTOR('',#19881,1.5106066017178);
#5585=VECTOR('',#19884,1.);
#5586=VECTOR('',#19889,0.72);
#5587=VECTOR('',#19896,1.);
#5588=VECTOR('',#19903,1.);
#6653=VERTEX_POINT('',#26836);
#6654=VERTEX_POINT('',#26837);
#6655=VERTEX_POINT('',#26839);
#6656=VERTEX_POINT('',#26841);
#6657=VERTEX_POINT('',#26843);
#6658=VERTEX_POINT('',#26845);
#6659=VERTEX_POINT('',#26849);
#6660=VERTEX_POINT('',#26851);
#6661=VERTEX_POINT('',#26853);
#6662=VERTEX_POINT('',#26857);
#6663=VERTEX_POINT('',#26859);
#6664=VERTEX_POINT('',#26863);
#6665=VERTEX_POINT('',#26865);
#6666=VERTEX_POINT('',#26869);
#6667=VERTEX_POINT('',#26870);
#6668=VERTEX_POINT('',#26872);
#6669=VERTEX_POINT('',#26874);
#6670=VERTEX_POINT('',#26878);
#6671=VERTEX_POINT('',#26880);
#6672=VERTEX_POINT('',#26884);
#6673=VERTEX_POINT('',#26886);
#6674=VERTEX_POINT('',#26890);
#6675=VERTEX_POINT('',#26892);
#6676=VERTEX_POINT('',#26894);
#6677=VERTEX_POINT('',#27017);
#6678=VERTEX_POINT('',#27018);
#6679=VERTEX_POINT('',#27020);
#6680=VERTEX_POINT('',#27086);
#6681=VERTEX_POINT('',#27089);
#6682=VERTEX_POINT('',#27091);
#6683=VERTEX_POINT('',#27095);
#6684=VERTEX_POINT('',#27096);
#6685=VERTEX_POINT('',#27129);
#6686=VERTEX_POINT('',#27133);
#6687=VERTEX_POINT('',#27139);
#6688=VERTEX_POINT('',#27143);
#6689=VERTEX_POINT('',#27250);
#6690=VERTEX_POINT('',#27252);
#6691=VERTEX_POINT('',#27263);
#6692=VERTEX_POINT('',#27289);
#6693=VERTEX_POINT('',#27291);
#6694=VERTEX_POINT('',#27295);
#6695=VERTEX_POINT('',#27299);
#6696=VERTEX_POINT('',#27302);
#6697=VERTEX_POINT('',#27303);
#6698=VERTEX_POINT('',#27305);
#6699=VERTEX_POINT('',#27307);
#6700=VERTEX_POINT('',#27311);
#6701=VERTEX_POINT('',#27312);
#6702=VERTEX_POINT('',#27323);
#6703=VERTEX_POINT('',#27325);
#6704=VERTEX_POINT('',#27330);
#6705=VERTEX_POINT('',#27331);
#6706=VERTEX_POINT('',#27333);
#6707=VERTEX_POINT('',#27335);
#6708=VERTEX_POINT('',#27337);
#6709=VERTEX_POINT('',#27339);
#6710=VERTEX_POINT('',#27343);
#6711=VERTEX_POINT('',#27345);
#6712=VERTEX_POINT('',#27347);
#6713=VERTEX_POINT('',#27349);
#6714=VERTEX_POINT('',#27353);
#6715=VERTEX_POINT('',#27355);
#6716=VERTEX_POINT('',#27357);
#6717=VERTEX_POINT('',#27361);
#6718=VERTEX_POINT('',#27365);
#6719=VERTEX_POINT('',#27367);
#6720=VERTEX_POINT('',#27372);
#6721=VERTEX_POINT('',#27374);
#6722=VERTEX_POINT('',#27376);
#6723=VERTEX_POINT('',#27381);
#6724=VERTEX_POINT('',#27387);
#6725=VERTEX_POINT('',#27388);
#6726=VERTEX_POINT('',#27390);
#6727=VERTEX_POINT('',#27395);
#6728=VERTEX_POINT('',#27399);
#6729=VERTEX_POINT('',#27401);
#6730=VERTEX_POINT('',#27403);
#6731=VERTEX_POINT('',#27405);
#6732=VERTEX_POINT('',#27407);
#6733=VERTEX_POINT('',#27411);
#6734=VERTEX_POINT('',#27413);
#6735=VERTEX_POINT('',#27415);
#6736=VERTEX_POINT('',#27419);
#6737=VERTEX_POINT('',#27426);
#6738=VERTEX_POINT('',#27428);
#6739=VERTEX_POINT('',#27432);
#6740=VERTEX_POINT('',#27433);
#6741=VERTEX_POINT('',#27435);
#6742=VERTEX_POINT('',#27437);
#6743=VERTEX_POINT('',#27441);
#6744=VERTEX_POINT('',#27442);
#6745=VERTEX_POINT('',#27444);
#6746=VERTEX_POINT('',#27446);
#6747=VERTEX_POINT('',#27450);
#6748=VERTEX_POINT('',#27451);
#6749=VERTEX_POINT('',#27458);
#6750=VERTEX_POINT('',#27460);
#6751=VERTEX_POINT('',#27464);
#6752=VERTEX_POINT('',#27468);
#6753=VERTEX_POINT('',#27474);
#6754=VERTEX_POINT('',#27476);
#6755=VERTEX_POINT('',#27478);
#6756=VERTEX_POINT('',#27480);
#6757=VERTEX_POINT('',#27483);
#6758=VERTEX_POINT('',#27487);
#6759=VERTEX_POINT('',#27490);
#6760=VERTEX_POINT('',#27494);
#6761=VERTEX_POINT('',#27498);
#6762=VERTEX_POINT('',#27502);
#6763=VERTEX_POINT('',#27513);
#6764=VERTEX_POINT('',#27517);
#6765=VERTEX_POINT('',#27521);
#6766=VERTEX_POINT('',#27525);
#6767=VERTEX_POINT('',#27526);
#6768=VERTEX_POINT('',#27528);
#6769=VERTEX_POINT('',#27530);
#6770=VERTEX_POINT('',#27533);
#6771=VERTEX_POINT('',#27535);
#6772=VERTEX_POINT('',#27553);
#6773=VERTEX_POINT('',#27557);
#6774=VERTEX_POINT('',#27561);
#6775=VERTEX_POINT('',#27565);
#8528=EDGE_CURVE('',#6653,#6654,#4211,.T.);
#8529=EDGE_CURVE('',#6654,#6655,#4212,.T.);
#8530=EDGE_CURVE('',#6655,#6656,#4213,.T.);
#8531=EDGE_CURVE('',#6656,#6657,#4214,.T.);
#8532=EDGE_CURVE('',#6657,#6658,#4215,.T.);
#8533=EDGE_CURVE('',#6658,#6653,#4216,.T.);
#8534=EDGE_CURVE('',#6659,#6656,#4217,.T.);
#8535=EDGE_CURVE('',#6659,#6660,#4218,.T.);
#8536=EDGE_CURVE('',#6661,#6660,#4219,.T.);
#8537=EDGE_CURVE('',#6661,#6657,#4220,.T.);
#8538=EDGE_CURVE('',#6655,#6662,#4221,.T.);
#8539=EDGE_CURVE('',#6662,#6663,#4222,.T.);
#8540=EDGE_CURVE('',#6663,#6659,#4223,.T.);
#8541=EDGE_CURVE('',#6664,#6654,#4224,.T.);
#8542=EDGE_CURVE('',#6665,#6664,#4225,.T.);
#8543=EDGE_CURVE('',#6655,#6665,#4226,.T.);
#8544=EDGE_CURVE('',#6666,#6667,#4227,.T.);
#8545=EDGE_CURVE('',#6667,#6668,#4228,.T.);
#8546=EDGE_CURVE('',#6668,#6669,#4229,.T.);
#8547=EDGE_CURVE('',#6669,#6666,#4230,.T.);
#8548=EDGE_CURVE('',#6667,#6670,#4231,.T.);
#8549=EDGE_CURVE('',#6670,#6671,#4232,.T.);
#8550=EDGE_CURVE('',#6671,#6668,#4233,.T.);
#8551=EDGE_CURVE('',#6669,#6672,#4234,.T.);
#8552=EDGE_CURVE('',#6672,#6673,#4235,.T.);
#8553=EDGE_CURVE('',#6673,#6666,#4236,.T.);
#8554=EDGE_CURVE('',#6674,#6673,#4237,.T.);
#8555=EDGE_CURVE('',#6674,#6675,#1410,.T.);
#8556=EDGE_CURVE('',#6675,#6676,#1411,.T.);
#8557=EDGE_CURVE('',#6670,#6676,#4238,.T.);
#8558=EDGE_CURVE('',#6677,#6678,#4239,.T.);
#8559=EDGE_CURVE('',#6678,#6679,#619,.T.);
#8560=EDGE_CURVE('',#6679,#6678,#620,.T.);
#8561=EDGE_CURVE('',#6677,#6677,#621,.T.);
#8562=EDGE_CURVE('',#6680,#6680,#1412,.T.);
#8563=EDGE_CURVE('',#6680,#6675,#4240,.T.);
#8564=EDGE_CURVE('',#6681,#6674,#96,.T.);
#8565=EDGE_CURVE('',#6682,#6681,#1413,.T.);
#8566=EDGE_CURVE('',#6676,#6682,#97,.T.);
#8567=EDGE_CURVE('',#6683,#6684,#622,.T.);
#8568=EDGE_CURVE('',#6684,#6683,#623,.T.);
#8569=EDGE_CURVE('',#6684,#6679,#4241,.T.);
#8570=EDGE_CURVE('',#6681,#6685,#130,.F.);
#8571=EDGE_CURVE('',#6685,#6686,#1414,.T.);
#8572=EDGE_CURVE('',#6682,#6686,#131,.T.);
#8573=EDGE_CURVE('',#6687,#6687,#1415,.T.);
#8574=EDGE_CURVE('',#6687,#6680,#4242,.T.);
#8575=EDGE_CURVE('',#6688,#6688,#1416,.T.);
#8576=EDGE_CURVE('',#6688,#6687,#4243,.T.);
#8577=EDGE_CURVE('',#6689,#6683,#4244,.T.);
#8578=EDGE_CURVE('',#6689,#6690,#624,.T.);
#8579=EDGE_CURVE('',#6690,#6691,#625,.T.);
#8580=EDGE_CURVE('',#6691,#6689,#626,.T.);
#8581=EDGE_CURVE('',#6692,#6692,#1417,.T.);
#8582=EDGE_CURVE('',#6692,#6693,#4245,.T.);
#8583=EDGE_CURVE('',#6693,#6693,#1418,.T.);
#8584=EDGE_CURVE('',#6688,#6694,#4246,.T.);
#8585=EDGE_CURVE('',#6694,#6694,#1419,.T.);
#8586=EDGE_CURVE('',#6695,#6695,#1420,.T.);
#8587=EDGE_CURVE('',#6696,#6697,#4247,.T.);
#8588=EDGE_CURVE('',#6697,#6698,#4248,.T.);
#8589=EDGE_CURVE('',#6698,#6699,#4249,.T.);
#8590=EDGE_CURVE('',#6699,#6696,#4250,.T.);
#8591=EDGE_CURVE('',#6700,#6701,#4251,.T.);
#8592=EDGE_CURVE('',#6701,#6665,#4252,.T.);
#8593=EDGE_CURVE('',#6664,#6700,#4253,.T.);
#8594=EDGE_CURVE('',#6697,#6665,#4254,.T.);
#8595=EDGE_CURVE('',#6701,#6698,#4255,.T.);
#8596=EDGE_CURVE('',#6664,#6696,#4256,.T.);
#8597=EDGE_CURVE('',#6699,#6700,#4257,.T.);
#8598=EDGE_CURVE('',#6702,#6654,#4258,.T.);
#8599=EDGE_CURVE('',#6703,#6702,#4259,.T.);
#8600=EDGE_CURVE('',#6703,#6696,#4260,.T.);
#8601=EDGE_CURVE('',#6704,#6705,#4261,.T.);
#8602=EDGE_CURVE('',#6705,#6706,#4262,.T.);
#8603=EDGE_CURVE('',#6706,#6707,#4263,.T.);
#8604=EDGE_CURVE('',#6707,#6708,#4264,.T.);
#8605=EDGE_CURVE('',#6708,#6709,#4265,.T.);
#8606=EDGE_CURVE('',#6709,#6704,#4266,.T.);
#8607=EDGE_CURVE('',#6704,#6710,#4267,.T.);
#8608=EDGE_CURVE('',#6710,#6711,#4268,.T.);
#8609=EDGE_CURVE('',#6711,#6712,#4269,.T.);
#8610=EDGE_CURVE('',#6712,#6713,#4270,.T.);
#8611=EDGE_CURVE('',#6713,#6705,#4271,.T.);
#8612=EDGE_CURVE('',#6709,#6714,#4272,.T.);
#8613=EDGE_CURVE('',#6715,#6714,#4273,.T.);
#8614=EDGE_CURVE('',#6716,#6715,#4274,.T.);
#8615=EDGE_CURVE('',#6710,#6716,#4275,.T.);
#8616=EDGE_CURVE('',#6717,#6708,#4276,.T.);
#8617=EDGE_CURVE('',#6714,#6717,#4277,.T.);
#8618=EDGE_CURVE('',#6662,#6718,#4278,.T.);
#8619=EDGE_CURVE('',#6718,#6719,#4279,.T.);
#8620=EDGE_CURVE('',#6719,#6663,#4280,.T.);
#8621=EDGE_CURVE('',#6706,#6719,#4281,.T.);
#8622=EDGE_CURVE('',#6720,#6718,#4282,.T.);
#8623=EDGE_CURVE('',#6720,#6721,#4283,.T.);
#8624=EDGE_CURVE('',#6722,#6721,#4284,.T.);
#8625=EDGE_CURVE('',#6722,#6707,#4285,.T.);
#8626=EDGE_CURVE('',#6671,#6720,#4286,.T.);
#8627=EDGE_CURVE('',#6662,#6723,#4287,.T.);
#8628=EDGE_CURVE('',#6723,#6668,#4288,.T.);
#8629=EDGE_CURVE('',#6697,#6723,#4289,.T.);
#8630=EDGE_CURVE('',#6724,#6725,#4290,.T.);
#8631=EDGE_CURVE('',#6725,#6726,#4291,.T.);
#8632=EDGE_CURVE('',#6726,#6702,#4292,.T.);
#8633=EDGE_CURVE('',#6702,#6724,#4293,.T.);
#8634=EDGE_CURVE('',#6653,#6727,#4294,.T.);
#8635=EDGE_CURVE('',#6727,#6724,#4295,.T.);
#8636=EDGE_CURVE('',#6725,#6728,#4296,.T.);
#8637=EDGE_CURVE('',#6729,#6728,#4297,.T.);
#8638=EDGE_CURVE('',#6729,#6730,#4298,.T.);
#8639=EDGE_CURVE('',#6731,#6730,#4299,.T.);
#8640=EDGE_CURVE('',#6731,#6732,#4300,.T.);
#8641=EDGE_CURVE('',#6726,#6732,#4301,.T.);
#8642=EDGE_CURVE('',#6733,#6727,#4302,.T.);
#8643=EDGE_CURVE('',#6734,#6733,#1421,.T.);
#8644=EDGE_CURVE('',#6735,#6734,#4303,.T.);
#8645=EDGE_CURVE('',#6728,#6735,#4304,.T.);
#8646=EDGE_CURVE('',#6658,#6736,#4305,.T.);
#8647=EDGE_CURVE('',#6736,#6733,#4306,.T.);
#8648=EDGE_CURVE('',#6735,#6715,#4307,.T.);
#8649=EDGE_CURVE('',#6717,#6729,#4308,.T.);
#8650=EDGE_CURVE('',#6737,#6734,#4309,.T.);
#8651=EDGE_CURVE('',#6737,#6738,#4310,.T.);
#8652=EDGE_CURVE('',#6738,#6716,#4311,.T.);
#8653=EDGE_CURVE('',#6739,#6740,#4312,.T.);
#8654=EDGE_CURVE('',#6740,#6741,#4313,.T.);
#8655=EDGE_CURVE('',#6741,#6742,#4314,.T.);
#8656=EDGE_CURVE('',#6742,#6739,#4315,.T.);
#8657=EDGE_CURVE('',#6743,#6744,#4316,.T.);
#8658=EDGE_CURVE('',#6744,#6745,#4317,.T.);
#8659=EDGE_CURVE('',#6745,#6746,#4318,.T.);
#8660=EDGE_CURVE('',#6746,#6743,#4319,.T.);
#8661=EDGE_CURVE('',#6747,#6748,#4320,.T.);
#8662=EDGE_CURVE('',#6748,#6745,#4321,.T.);
#8663=EDGE_CURVE('',#6744,#6739,#4322,.T.);
#8664=EDGE_CURVE('',#6742,#6747,#4323,.T.);
#8665=EDGE_CURVE('',#6740,#6743,#4324,.T.);
#8666=EDGE_CURVE('',#6746,#6749,#4325,.T.);
#8667=EDGE_CURVE('',#6749,#6750,#4326,.T.);
#8668=EDGE_CURVE('',#6750,#6741,#4327,.T.);
#8669=EDGE_CURVE('',#6751,#6749,#4328,.T.);
#8670=EDGE_CURVE('',#6750,#6751,#4329,.T.);
#8671=EDGE_CURVE('',#6752,#6748,#4330,.T.);
#8672=EDGE_CURVE('',#6752,#6751,#4331,.T.);
#8673=EDGE_CURVE('',#6712,#6737,#4332,.T.);
#8674=EDGE_CURVE('',#6738,#6711,#4333,.T.);
#8675=EDGE_CURVE('',#6753,#6753,#1422,.T.);
#8676=EDGE_CURVE('',#6754,#6754,#1423,.T.);
#8677=EDGE_CURVE('',#6755,#6755,#1424,.T.);
#8678=EDGE_CURVE('',#6756,#6756,#1425,.T.);
#8679=EDGE_CURVE('',#6753,#6757,#4334,.T.);
#8680=EDGE_CURVE('',#6757,#6757,#1426,.T.);
#8681=EDGE_CURVE('',#6758,#6757,#4335,.T.);
#8682=EDGE_CURVE('',#6756,#6759,#4336,.T.);
#8683=EDGE_CURVE('',#6759,#6759,#1427,.T.);
#8684=EDGE_CURVE('',#6759,#6760,#4337,.T.);
#8685=EDGE_CURVE('',#6760,#6760,#1428,.T.);
#8686=EDGE_CURVE('',#6754,#6761,#4338,.T.);
#8687=EDGE_CURVE('',#6761,#6761,#1429,.T.);
#8688=EDGE_CURVE('',#6761,#6762,#4339,.T.);
#8689=EDGE_CURVE('',#6762,#6762,#1430,.T.);
#8690=EDGE_CURVE('',#6736,#6737,#1431,.T.);
#8691=EDGE_CURVE('',#6712,#6661,#1432,.T.);
#8692=EDGE_CURVE('',#6660,#6713,#1433,.T.);
#8693=EDGE_CURVE('',#6763,#6763,#1434,.T.);
#8694=EDGE_CURVE('',#6763,#6755,#4340,.T.);
#8695=EDGE_CURVE('',#6763,#6764,#4341,.T.);
#8696=EDGE_CURVE('',#6764,#6764,#1435,.T.);
#8697=EDGE_CURVE('',#6765,#6765,#1436,.T.);
#8698=EDGE_CURVE('',#6765,#6760,#4342,.T.);
#8699=EDGE_CURVE('',#6766,#6767,#4343,.T.);
#8700=EDGE_CURVE('',#6768,#6766,#4344,.T.);
#8701=EDGE_CURVE('',#6769,#6768,#4345,.T.);
#8702=EDGE_CURVE('',#6767,#6769,#4346,.T.);
#8703=EDGE_CURVE('',#6770,#6770,#1437,.T.);
#8704=EDGE_CURVE('',#6771,#6771,#1438,.T.);
#8705=EDGE_CURVE('',#6770,#6762,#4347,.T.);
#8706=EDGE_CURVE('',#6730,#6722,#4348,.T.);
#8707=EDGE_CURVE('',#6722,#6769,#4349,.T.);
#8708=EDGE_CURVE('',#6768,#6730,#4350,.T.);
#8709=EDGE_CURVE('',#6767,#6721,#4351,.T.);
#8710=EDGE_CURVE('',#6721,#6731,#4352,.T.);
#8711=EDGE_CURVE('',#6731,#6766,#4353,.T.);
#8712=EDGE_CURVE('',#6686,#6685,#4354,.T.);
#8713=EDGE_CURVE('',#6732,#6672,#4355,.T.);
#8714=EDGE_CURVE('',#6764,#6772,#4356,.T.);
#8715=EDGE_CURVE('',#6772,#6772,#1439,.T.);
#8716=EDGE_CURVE('',#6773,#6773,#1440,.T.);
#8717=EDGE_CURVE('',#6773,#6772,#4357,.T.);
#8718=EDGE_CURVE('',#6774,#6774,#1441,.T.);
#8719=EDGE_CURVE('',#6774,#6771,#4358,.T.);
#8720=EDGE_CURVE('',#6774,#6775,#4359,.T.);
#8721=EDGE_CURVE('',#6775,#6775,#1442,.T.);
#8722=EDGE_CURVE('',#6775,#6773,#4360,.T.);
#8723=EDGE_CURVE('',#6747,#6752,#4361,.T.);
#8724=EDGE_CURVE('',#6695,#6692,#4362,.T.);
#8725=EDGE_CURVE('',#6669,#6703,#4363,.T.);
#8726=EDGE_CURVE('',#6736,#6661,#4364,.T.);
#11825=ORIENTED_EDGE('',*,*,#8528,.T.);
#11826=ORIENTED_EDGE('',*,*,#8529,.T.);
#11827=ORIENTED_EDGE('',*,*,#8530,.T.);
#11828=ORIENTED_EDGE('',*,*,#8531,.T.);
#11829=ORIENTED_EDGE('',*,*,#8532,.T.);
#11830=ORIENTED_EDGE('',*,*,#8533,.T.);
#11831=ORIENTED_EDGE('',*,*,#8531,.F.);
#11832=ORIENTED_EDGE('',*,*,#8534,.F.);
#11833=ORIENTED_EDGE('',*,*,#8535,.T.);
#11834=ORIENTED_EDGE('',*,*,#8536,.F.);
#11835=ORIENTED_EDGE('',*,*,#8537,.T.);
#11836=ORIENTED_EDGE('',*,*,#8530,.F.);
#11837=ORIENTED_EDGE('',*,*,#8538,.T.);
#11838=ORIENTED_EDGE('',*,*,#8539,.T.);
#11839=ORIENTED_EDGE('',*,*,#8540,.T.);
#11840=ORIENTED_EDGE('',*,*,#8534,.T.);
#11841=ORIENTED_EDGE('',*,*,#8529,.F.);
#11842=ORIENTED_EDGE('',*,*,#8541,.F.);
#11843=ORIENTED_EDGE('',*,*,#8542,.F.);
#11844=ORIENTED_EDGE('',*,*,#8543,.F.);
#11845=ORIENTED_EDGE('',*,*,#8544,.T.);
#11846=ORIENTED_EDGE('',*,*,#8545,.T.);
#11847=ORIENTED_EDGE('',*,*,#8546,.T.);
#11848=ORIENTED_EDGE('',*,*,#8547,.T.);
#11849=ORIENTED_EDGE('',*,*,#8548,.T.);
#11850=ORIENTED_EDGE('',*,*,#8549,.T.);
#11851=ORIENTED_EDGE('',*,*,#8550,.T.);
#11852=ORIENTED_EDGE('',*,*,#8545,.F.);
#11853=ORIENTED_EDGE('',*,*,#8551,.T.);
#11854=ORIENTED_EDGE('',*,*,#8552,.T.);
#11855=ORIENTED_EDGE('',*,*,#8553,.T.);
#11856=ORIENTED_EDGE('',*,*,#8547,.F.);
#11857=ORIENTED_EDGE('',*,*,#8548,.F.);
#11858=ORIENTED_EDGE('',*,*,#8544,.F.);
#11859=ORIENTED_EDGE('',*,*,#8553,.F.);
#11860=ORIENTED_EDGE('',*,*,#8554,.F.);
#11861=ORIENTED_EDGE('',*,*,#8555,.T.);
#11862=ORIENTED_EDGE('',*,*,#8556,.T.);
#11863=ORIENTED_EDGE('',*,*,#8557,.F.);
#11864=ORIENTED_EDGE('',*,*,#8558,.T.);
#11865=ORIENTED_EDGE('',*,*,#8559,.T.);
#11866=ORIENTED_EDGE('',*,*,#8560,.T.);
#11867=ORIENTED_EDGE('',*,*,#8558,.F.);
#11868=ORIENTED_EDGE('',*,*,#8561,.T.);
#11869=ORIENTED_EDGE('',*,*,#8562,.F.);
#11870=ORIENTED_EDGE('',*,*,#8563,.T.);
#11871=ORIENTED_EDGE('',*,*,#8555,.F.);
#11872=ORIENTED_EDGE('',*,*,#8564,.F.);
#11873=ORIENTED_EDGE('',*,*,#8565,.F.);
#11874=ORIENTED_EDGE('',*,*,#8566,.F.);
#11875=ORIENTED_EDGE('',*,*,#8556,.F.);
#11876=ORIENTED_EDGE('',*,*,#8563,.F.);
#11877=ORIENTED_EDGE('',*,*,#8561,.F.);
#11878=ORIENTED_EDGE('',*,*,#8567,.F.);
#11879=ORIENTED_EDGE('',*,*,#8568,.F.);
#11880=ORIENTED_EDGE('',*,*,#8569,.T.);
#11881=ORIENTED_EDGE('',*,*,#8559,.F.);
#11882=ORIENTED_EDGE('',*,*,#8560,.F.);
#11883=ORIENTED_EDGE('',*,*,#8569,.F.);
#11884=ORIENTED_EDGE('',*,*,#8570,.T.);
#11885=ORIENTED_EDGE('',*,*,#8571,.T.);
#11886=ORIENTED_EDGE('',*,*,#8572,.F.);
#11887=ORIENTED_EDGE('',*,*,#8565,.T.);
#11888=ORIENTED_EDGE('',*,*,#8573,.T.);
#11889=ORIENTED_EDGE('',*,*,#8574,.T.);
#11890=ORIENTED_EDGE('',*,*,#8562,.T.);
#11891=ORIENTED_EDGE('',*,*,#8574,.F.);
#11892=ORIENTED_EDGE('',*,*,#8575,.F.);
#11893=ORIENTED_EDGE('',*,*,#8576,.T.);
#11894=ORIENTED_EDGE('',*,*,#8573,.F.);
#11895=ORIENTED_EDGE('',*,*,#8576,.F.);
#11896=ORIENTED_EDGE('',*,*,#8577,.T.);
#11897=ORIENTED_EDGE('',*,*,#8567,.T.);
#11898=ORIENTED_EDGE('',*,*,#8568,.T.);
#11899=ORIENTED_EDGE('',*,*,#8577,.F.);
#11900=ORIENTED_EDGE('',*,*,#8578,.T.);
#11901=ORIENTED_EDGE('',*,*,#8579,.T.);
#11902=ORIENTED_EDGE('',*,*,#8580,.T.);
#11903=ORIENTED_EDGE('',*,*,#8581,.F.);
#11904=ORIENTED_EDGE('',*,*,#8582,.T.);
#11905=ORIENTED_EDGE('',*,*,#8583,.T.);
#11906=ORIENTED_EDGE('',*,*,#8582,.F.);
#11907=ORIENTED_EDGE('',*,*,#8580,.F.);
#11908=ORIENTED_EDGE('',*,*,#8579,.F.);
#11909=ORIENTED_EDGE('',*,*,#8578,.F.);
#11910=ORIENTED_EDGE('',*,*,#8575,.T.);
#11911=ORIENTED_EDGE('',*,*,#8584,.T.);
#11912=ORIENTED_EDGE('',*,*,#8585,.T.);
#11913=ORIENTED_EDGE('',*,*,#8584,.F.);
#11914=ORIENTED_EDGE('',*,*,#8585,.F.);
#11915=ORIENTED_EDGE('',*,*,#8586,.F.);
#11916=ORIENTED_EDGE('',*,*,#8587,.T.);
#11917=ORIENTED_EDGE('',*,*,#8588,.T.);
#11918=ORIENTED_EDGE('',*,*,#8589,.T.);
#11919=ORIENTED_EDGE('',*,*,#8590,.T.);
#11920=ORIENTED_EDGE('',*,*,#8591,.T.);
#11921=ORIENTED_EDGE('',*,*,#8592,.T.);
#11922=ORIENTED_EDGE('',*,*,#8542,.T.);
#11923=ORIENTED_EDGE('',*,*,#8593,.T.);
#11924=ORIENTED_EDGE('',*,*,#8594,.T.);
#11925=ORIENTED_EDGE('',*,*,#8592,.F.);
#11926=ORIENTED_EDGE('',*,*,#8595,.T.);
#11927=ORIENTED_EDGE('',*,*,#8588,.F.);
#11928=ORIENTED_EDGE('',*,*,#8596,.T.);
#11929=ORIENTED_EDGE('',*,*,#8590,.F.);
#11930=ORIENTED_EDGE('',*,*,#8597,.T.);
#11931=ORIENTED_EDGE('',*,*,#8593,.F.);
#11932=ORIENTED_EDGE('',*,*,#8596,.F.);
#11933=ORIENTED_EDGE('',*,*,#8541,.T.);
#11934=ORIENTED_EDGE('',*,*,#8598,.F.);
#11935=ORIENTED_EDGE('',*,*,#8599,.F.);
#11936=ORIENTED_EDGE('',*,*,#8600,.T.);
#11937=ORIENTED_EDGE('',*,*,#8591,.F.);
#11938=ORIENTED_EDGE('',*,*,#8597,.F.);
#11939=ORIENTED_EDGE('',*,*,#8589,.F.);
#11940=ORIENTED_EDGE('',*,*,#8595,.F.);
#11941=ORIENTED_EDGE('',*,*,#8601,.T.);
#11942=ORIENTED_EDGE('',*,*,#8602,.T.);
#11943=ORIENTED_EDGE('',*,*,#8603,.T.);
#11944=ORIENTED_EDGE('',*,*,#8604,.T.);
#11945=ORIENTED_EDGE('',*,*,#8605,.T.);
#11946=ORIENTED_EDGE('',*,*,#8606,.T.);
#11947=ORIENTED_EDGE('',*,*,#8601,.F.);
#11948=ORIENTED_EDGE('',*,*,#8607,.T.);
#11949=ORIENTED_EDGE('',*,*,#8608,.T.);
#11950=ORIENTED_EDGE('',*,*,#8609,.T.);
#11951=ORIENTED_EDGE('',*,*,#8610,.T.);
#11952=ORIENTED_EDGE('',*,*,#8611,.T.);
#11953=ORIENTED_EDGE('',*,*,#8606,.F.);
#11954=ORIENTED_EDGE('',*,*,#8612,.T.);
#11955=ORIENTED_EDGE('',*,*,#8613,.F.);
#11956=ORIENTED_EDGE('',*,*,#8614,.F.);
#11957=ORIENTED_EDGE('',*,*,#8615,.F.);
#11958=ORIENTED_EDGE('',*,*,#8607,.F.);
#11959=ORIENTED_EDGE('',*,*,#8605,.F.);
#11960=ORIENTED_EDGE('',*,*,#8616,.F.);
#11961=ORIENTED_EDGE('',*,*,#8617,.F.);
#11962=ORIENTED_EDGE('',*,*,#8612,.F.);
#11963=ORIENTED_EDGE('',*,*,#8618,.T.);
#11964=ORIENTED_EDGE('',*,*,#8619,.T.);
#11965=ORIENTED_EDGE('',*,*,#8620,.T.);
#11966=ORIENTED_EDGE('',*,*,#8539,.F.);
#11967=ORIENTED_EDGE('',*,*,#8603,.F.);
#11968=ORIENTED_EDGE('',*,*,#8621,.T.);
#11969=ORIENTED_EDGE('',*,*,#8619,.F.);
#11970=ORIENTED_EDGE('',*,*,#8622,.F.);
#11971=ORIENTED_EDGE('',*,*,#8623,.T.);
#11972=ORIENTED_EDGE('',*,*,#8624,.F.);
#11973=ORIENTED_EDGE('',*,*,#8625,.T.);
#11974=ORIENTED_EDGE('',*,*,#8550,.F.);
#11975=ORIENTED_EDGE('',*,*,#8626,.T.);
#11976=ORIENTED_EDGE('',*,*,#8622,.T.);
#11977=ORIENTED_EDGE('',*,*,#8618,.F.);
#11978=ORIENTED_EDGE('',*,*,#8627,.T.);
#11979=ORIENTED_EDGE('',*,*,#8628,.T.);
#11980=ORIENTED_EDGE('',*,*,#8594,.F.);
#11981=ORIENTED_EDGE('',*,*,#8629,.T.);
#11982=ORIENTED_EDGE('',*,*,#8627,.F.);
#11983=ORIENTED_EDGE('',*,*,#8538,.F.);
#11984=ORIENTED_EDGE('',*,*,#8543,.T.);
#11985=ORIENTED_EDGE('',*,*,#8630,.T.);
#11986=ORIENTED_EDGE('',*,*,#8631,.T.);
#11987=ORIENTED_EDGE('',*,*,#8632,.T.);
#11988=ORIENTED_EDGE('',*,*,#8633,.T.);
#11989=ORIENTED_EDGE('',*,*,#8528,.F.);
#11990=ORIENTED_EDGE('',*,*,#8634,.T.);
#11991=ORIENTED_EDGE('',*,*,#8635,.T.);
#11992=ORIENTED_EDGE('',*,*,#8633,.F.);
#11993=ORIENTED_EDGE('',*,*,#8598,.T.);
#11994=ORIENTED_EDGE('',*,*,#8631,.F.);
#11995=ORIENTED_EDGE('',*,*,#8636,.T.);
#11996=ORIENTED_EDGE('',*,*,#8637,.F.);
#11997=ORIENTED_EDGE('',*,*,#8638,.T.);
#11998=ORIENTED_EDGE('',*,*,#8639,.F.);
#11999=ORIENTED_EDGE('',*,*,#8640,.T.);
#12000=ORIENTED_EDGE('',*,*,#8641,.F.);
#12001=ORIENTED_EDGE('',*,*,#8630,.F.);
#12002=ORIENTED_EDGE('',*,*,#8635,.F.);
#12003=ORIENTED_EDGE('',*,*,#8642,.F.);
#12004=ORIENTED_EDGE('',*,*,#8643,.F.);
#12005=ORIENTED_EDGE('',*,*,#8644,.F.);
#12006=ORIENTED_EDGE('',*,*,#8645,.F.);
#12007=ORIENTED_EDGE('',*,*,#8636,.F.);
#12008=ORIENTED_EDGE('',*,*,#8533,.F.);
#12009=ORIENTED_EDGE('',*,*,#8646,.T.);
#12010=ORIENTED_EDGE('',*,*,#8647,.T.);
#12011=ORIENTED_EDGE('',*,*,#8642,.T.);
#12012=ORIENTED_EDGE('',*,*,#8634,.F.);
#12013=ORIENTED_EDGE('',*,*,#8637,.T.);
#12014=ORIENTED_EDGE('',*,*,#8645,.T.);
#12015=ORIENTED_EDGE('',*,*,#8648,.T.);
#12016=ORIENTED_EDGE('',*,*,#8613,.T.);
#12017=ORIENTED_EDGE('',*,*,#8617,.T.);
#12018=ORIENTED_EDGE('',*,*,#8649,.T.);
#12019=ORIENTED_EDGE('',*,*,#8648,.F.);
#12020=ORIENTED_EDGE('',*,*,#8644,.T.);
#12021=ORIENTED_EDGE('',*,*,#8650,.F.);
#12022=ORIENTED_EDGE('',*,*,#8651,.T.);
#12023=ORIENTED_EDGE('',*,*,#8652,.T.);
#12024=ORIENTED_EDGE('',*,*,#8614,.T.);
#12025=ORIENTED_EDGE('',*,*,#8653,.T.);
#12026=ORIENTED_EDGE('',*,*,#8654,.T.);
#12027=ORIENTED_EDGE('',*,*,#8655,.T.);
#12028=ORIENTED_EDGE('',*,*,#8656,.T.);
#12029=ORIENTED_EDGE('',*,*,#8657,.T.);
#12030=ORIENTED_EDGE('',*,*,#8658,.T.);
#12031=ORIENTED_EDGE('',*,*,#8659,.T.);
#12032=ORIENTED_EDGE('',*,*,#8660,.T.);
#12033=ORIENTED_EDGE('',*,*,#8661,.T.);
#12034=ORIENTED_EDGE('',*,*,#8662,.T.);
#12035=ORIENTED_EDGE('',*,*,#8658,.F.);
#12036=ORIENTED_EDGE('',*,*,#8663,.T.);
#12037=ORIENTED_EDGE('',*,*,#8656,.F.);
#12038=ORIENTED_EDGE('',*,*,#8664,.T.);
#12039=ORIENTED_EDGE('',*,*,#8665,.T.);
#12040=ORIENTED_EDGE('',*,*,#8660,.F.);
#12041=ORIENTED_EDGE('',*,*,#8666,.T.);
#12042=ORIENTED_EDGE('',*,*,#8667,.T.);
#12043=ORIENTED_EDGE('',*,*,#8668,.T.);
#12044=ORIENTED_EDGE('',*,*,#8654,.F.);
#12045=ORIENTED_EDGE('',*,*,#8667,.F.);
#12046=ORIENTED_EDGE('',*,*,#8669,.F.);
#12047=ORIENTED_EDGE('',*,*,#8670,.F.);
#12048=ORIENTED_EDGE('',*,*,#8659,.F.);
#12049=ORIENTED_EDGE('',*,*,#8662,.F.);
#12050=ORIENTED_EDGE('',*,*,#8671,.F.);
#12051=ORIENTED_EDGE('',*,*,#8672,.T.);
#12052=ORIENTED_EDGE('',*,*,#8669,.T.);
#12053=ORIENTED_EDGE('',*,*,#8666,.F.);
#12054=ORIENTED_EDGE('',*,*,#8651,.F.);
#12055=ORIENTED_EDGE('',*,*,#8673,.F.);
#12056=ORIENTED_EDGE('',*,*,#8609,.F.);
#12057=ORIENTED_EDGE('',*,*,#8674,.F.);
#12058=ORIENTED_EDGE('',*,*,#8675,.F.);
#12059=ORIENTED_EDGE('',*,*,#8676,.F.);
#12060=ORIENTED_EDGE('',*,*,#8677,.F.);
#12061=ORIENTED_EDGE('',*,*,#8678,.F.);
#12062=ORIENTED_EDGE('',*,*,#8657,.F.);
#12063=ORIENTED_EDGE('',*,*,#8665,.F.);
#12064=ORIENTED_EDGE('',*,*,#8653,.F.);
#12065=ORIENTED_EDGE('',*,*,#8663,.F.);
#12066=ORIENTED_EDGE('',*,*,#8675,.T.);
#12067=ORIENTED_EDGE('',*,*,#8679,.T.);
#12068=ORIENTED_EDGE('',*,*,#8680,.T.);
#12069=ORIENTED_EDGE('',*,*,#8679,.F.);
#12070=ORIENTED_EDGE('',*,*,#8681,.T.);
#12071=ORIENTED_EDGE('',*,*,#8680,.F.);
#12072=ORIENTED_EDGE('',*,*,#8681,.F.);
#12073=ORIENTED_EDGE('',*,*,#8678,.T.);
#12074=ORIENTED_EDGE('',*,*,#8682,.T.);
#12075=ORIENTED_EDGE('',*,*,#8683,.T.);
#12076=ORIENTED_EDGE('',*,*,#8682,.F.);
#12077=ORIENTED_EDGE('',*,*,#8683,.F.);
#12078=ORIENTED_EDGE('',*,*,#8684,.T.);
#12079=ORIENTED_EDGE('',*,*,#8685,.F.);
#12080=ORIENTED_EDGE('',*,*,#8684,.F.);
#12081=ORIENTED_EDGE('',*,*,#8676,.T.);
#12082=ORIENTED_EDGE('',*,*,#8686,.T.);
#12083=ORIENTED_EDGE('',*,*,#8687,.T.);
#12084=ORIENTED_EDGE('',*,*,#8686,.F.);
#12085=ORIENTED_EDGE('',*,*,#8687,.F.);
#12086=ORIENTED_EDGE('',*,*,#8688,.T.);
#12087=ORIENTED_EDGE('',*,*,#8689,.F.);
#12088=ORIENTED_EDGE('',*,*,#8688,.F.);
#12089=ORIENTED_EDGE('',*,*,#8647,.F.);
#12090=ORIENTED_EDGE('',*,*,#8690,.T.);
#12091=ORIENTED_EDGE('',*,*,#8650,.T.);
#12092=ORIENTED_EDGE('',*,*,#8643,.T.);
#12093=ORIENTED_EDGE('',*,*,#8615,.T.);
#12094=ORIENTED_EDGE('',*,*,#8652,.F.);
#12095=ORIENTED_EDGE('',*,*,#8674,.T.);
#12096=ORIENTED_EDGE('',*,*,#8608,.F.);
#12097=ORIENTED_EDGE('',*,*,#8610,.F.);
#12098=ORIENTED_EDGE('',*,*,#8691,.T.);
#12099=ORIENTED_EDGE('',*,*,#8536,.T.);
#12100=ORIENTED_EDGE('',*,*,#8692,.T.);
#12101=ORIENTED_EDGE('',*,*,#8602,.F.);
#12102=ORIENTED_EDGE('',*,*,#8611,.F.);
#12103=ORIENTED_EDGE('',*,*,#8692,.F.);
#12104=ORIENTED_EDGE('',*,*,#8535,.F.);
#12105=ORIENTED_EDGE('',*,*,#8540,.F.);
#12106=ORIENTED_EDGE('',*,*,#8620,.F.);
#12107=ORIENTED_EDGE('',*,*,#8621,.F.);
#12108=ORIENTED_EDGE('',*,*,#8693,.T.);
#12109=ORIENTED_EDGE('',*,*,#8694,.T.);
#12110=ORIENTED_EDGE('',*,*,#8677,.T.);
#12111=ORIENTED_EDGE('',*,*,#8694,.F.);
#12112=ORIENTED_EDGE('',*,*,#8693,.F.);
#12113=ORIENTED_EDGE('',*,*,#8695,.T.);
#12114=ORIENTED_EDGE('',*,*,#8696,.F.);
#12115=ORIENTED_EDGE('',*,*,#8695,.F.);
#12116=ORIENTED_EDGE('',*,*,#8697,.T.);
#12117=ORIENTED_EDGE('',*,*,#8698,.T.);
#12118=ORIENTED_EDGE('',*,*,#8685,.T.);
#12119=ORIENTED_EDGE('',*,*,#8698,.F.);
#12120=ORIENTED_EDGE('',*,*,#8699,.F.);
#12121=ORIENTED_EDGE('',*,*,#8700,.F.);
#12122=ORIENTED_EDGE('',*,*,#8701,.F.);
#12123=ORIENTED_EDGE('',*,*,#8702,.F.);
#12124=ORIENTED_EDGE('',*,*,#8703,.F.);
#12125=ORIENTED_EDGE('',*,*,#8704,.F.);
#12126=ORIENTED_EDGE('',*,*,#8697,.F.);
#12127=ORIENTED_EDGE('',*,*,#8703,.T.);
#12128=ORIENTED_EDGE('',*,*,#8705,.T.);
#12129=ORIENTED_EDGE('',*,*,#8689,.T.);
#12130=ORIENTED_EDGE('',*,*,#8705,.F.);
#12131=ORIENTED_EDGE('',*,*,#8706,.T.);
#12132=ORIENTED_EDGE('',*,*,#8707,.T.);
#12133=ORIENTED_EDGE('',*,*,#8701,.T.);
#12134=ORIENTED_EDGE('',*,*,#8708,.T.);
#12135=ORIENTED_EDGE('',*,*,#8699,.T.);
#12136=ORIENTED_EDGE('',*,*,#8709,.T.);
#12137=ORIENTED_EDGE('',*,*,#8710,.T.);
#12138=ORIENTED_EDGE('',*,*,#8711,.T.);
#12139=ORIENTED_EDGE('',*,*,#8624,.T.);
#12140=ORIENTED_EDGE('',*,*,#8709,.F.);
#12141=ORIENTED_EDGE('',*,*,#8702,.T.);
#12142=ORIENTED_EDGE('',*,*,#8707,.F.);
#12143=ORIENTED_EDGE('',*,*,#8639,.T.);
#12144=ORIENTED_EDGE('',*,*,#8708,.F.);
#12145=ORIENTED_EDGE('',*,*,#8700,.T.);
#12146=ORIENTED_EDGE('',*,*,#8711,.F.);
#12147=ORIENTED_EDGE('',*,*,#8549,.F.);
#12148=ORIENTED_EDGE('',*,*,#8557,.T.);
#12149=ORIENTED_EDGE('',*,*,#8566,.T.);
#12150=ORIENTED_EDGE('',*,*,#8572,.T.);
#12151=ORIENTED_EDGE('',*,*,#8712,.T.);
#12152=ORIENTED_EDGE('',*,*,#8570,.F.);
#12153=ORIENTED_EDGE('',*,*,#8564,.T.);
#12154=ORIENTED_EDGE('',*,*,#8554,.T.);
#12155=ORIENTED_EDGE('',*,*,#8552,.F.);
#12156=ORIENTED_EDGE('',*,*,#8713,.F.);
#12157=ORIENTED_EDGE('',*,*,#8640,.F.);
#12158=ORIENTED_EDGE('',*,*,#8710,.F.);
#12159=ORIENTED_EDGE('',*,*,#8623,.F.);
#12160=ORIENTED_EDGE('',*,*,#8626,.F.);
#12161=ORIENTED_EDGE('',*,*,#8696,.T.);
#12162=ORIENTED_EDGE('',*,*,#8714,.T.);
#12163=ORIENTED_EDGE('',*,*,#8715,.T.);
#12164=ORIENTED_EDGE('',*,*,#8714,.F.);
#12165=ORIENTED_EDGE('',*,*,#8716,.F.);
#12166=ORIENTED_EDGE('',*,*,#8717,.T.);
#12167=ORIENTED_EDGE('',*,*,#8715,.F.);
#12168=ORIENTED_EDGE('',*,*,#8717,.F.);
#12169=ORIENTED_EDGE('',*,*,#8718,.T.);
#12170=ORIENTED_EDGE('',*,*,#8719,.T.);
#12171=ORIENTED_EDGE('',*,*,#8704,.T.);
#12172=ORIENTED_EDGE('',*,*,#8719,.F.);
#12173=ORIENTED_EDGE('',*,*,#8718,.F.);
#12174=ORIENTED_EDGE('',*,*,#8720,.T.);
#12175=ORIENTED_EDGE('',*,*,#8721,.F.);
#12176=ORIENTED_EDGE('',*,*,#8720,.F.);
#12177=ORIENTED_EDGE('',*,*,#8721,.T.);
#12178=ORIENTED_EDGE('',*,*,#8722,.T.);
#12179=ORIENTED_EDGE('',*,*,#8716,.T.);
#12180=ORIENTED_EDGE('',*,*,#8722,.F.);
#12181=ORIENTED_EDGE('',*,*,#8655,.F.);
#12182=ORIENTED_EDGE('',*,*,#8668,.F.);
#12183=ORIENTED_EDGE('',*,*,#8670,.T.);
#12184=ORIENTED_EDGE('',*,*,#8672,.F.);
#12185=ORIENTED_EDGE('',*,*,#8723,.F.);
#12186=ORIENTED_EDGE('',*,*,#8664,.F.);
#12187=ORIENTED_EDGE('',*,*,#8661,.F.);
#12188=ORIENTED_EDGE('',*,*,#8723,.T.);
#12189=ORIENTED_EDGE('',*,*,#8671,.T.);
#12190=ORIENTED_EDGE('',*,*,#8586,.T.);
#12191=ORIENTED_EDGE('',*,*,#8724,.T.);
#12192=ORIENTED_EDGE('',*,*,#8581,.T.);
#12193=ORIENTED_EDGE('',*,*,#8724,.F.);
#12194=ORIENTED_EDGE('',*,*,#8583,.F.);
#12195=ORIENTED_EDGE('',*,*,#8571,.F.);
#12196=ORIENTED_EDGE('',*,*,#8712,.F.);
#12197=ORIENTED_EDGE('',*,*,#8546,.F.);
#12198=ORIENTED_EDGE('',*,*,#8628,.F.);
#12199=ORIENTED_EDGE('',*,*,#8629,.F.);
#12200=ORIENTED_EDGE('',*,*,#8587,.F.);
#12201=ORIENTED_EDGE('',*,*,#8600,.F.);
#12202=ORIENTED_EDGE('',*,*,#8725,.F.);
#12203=ORIENTED_EDGE('',*,*,#8551,.F.);
#12204=ORIENTED_EDGE('',*,*,#8725,.T.);
#12205=ORIENTED_EDGE('',*,*,#8599,.T.);
#12206=ORIENTED_EDGE('',*,*,#8632,.F.);
#12207=ORIENTED_EDGE('',*,*,#8641,.T.);
#12208=ORIENTED_EDGE('',*,*,#8713,.T.);
#12209=ORIENTED_EDGE('',*,*,#8604,.F.);
#12210=ORIENTED_EDGE('',*,*,#8625,.F.);
#12211=ORIENTED_EDGE('',*,*,#8706,.F.);
#12212=ORIENTED_EDGE('',*,*,#8638,.F.);
#12213=ORIENTED_EDGE('',*,*,#8649,.F.);
#12214=ORIENTED_EDGE('',*,*,#8616,.T.);
#12215=ORIENTED_EDGE('',*,*,#8532,.F.);
#12216=ORIENTED_EDGE('',*,*,#8537,.F.);
#12217=ORIENTED_EDGE('',*,*,#8726,.F.);
#12218=ORIENTED_EDGE('',*,*,#8646,.F.);
#12219=ORIENTED_EDGE('',*,*,#8690,.F.);
#12220=ORIENTED_EDGE('',*,*,#8726,.T.);
#12221=ORIENTED_EDGE('',*,*,#8691,.F.);
#12222=ORIENTED_EDGE('',*,*,#8673,.T.);
#15033=PLANE('',#16984);
#15034=PLANE('',#16985);
#15035=PLANE('',#16986);
#15036=PLANE('',#16987);
#15037=PLANE('',#16988);
#15038=PLANE('',#16989);
#15039=PLANE('',#16990);
#15040=PLANE('',#16991);
#15041=PLANE('',#17011);
#15042=PLANE('',#17013);
#15043=PLANE('',#17014);
#15044=PLANE('',#17015);
#15045=PLANE('',#17016);
#15046=PLANE('',#17017);
#15047=PLANE('',#17018);
#15048=PLANE('',#17019);
#15049=PLANE('',#17020);
#15050=PLANE('',#17021);
#15051=PLANE('',#17022);
#15052=PLANE('',#17023);
#15053=PLANE('',#17024);
#15054=PLANE('',#17025);
#15055=PLANE('',#17026);
#15056=PLANE('',#17027);
#15057=PLANE('',#17028);
#15058=PLANE('',#17029);
#15059=PLANE('',#17030);
#15060=PLANE('',#17032);
#15061=PLANE('',#17033);
#15062=PLANE('',#17034);
#15063=PLANE('',#17035);
#15064=PLANE('',#17036);
#15065=PLANE('',#17037);
#15066=PLANE('',#17038);
#15067=PLANE('',#17039);
#15068=PLANE('',#17040);
#15069=PLANE('',#17041);
#15070=PLANE('',#17059);
#15071=PLANE('',#17063);
#15072=PLANE('',#17070);
#15073=PLANE('',#17074);
#15074=PLANE('',#17075);
#15075=PLANE('',#17076);
#15076=PLANE('',#17077);
#15077=PLANE('',#17078);
#15078=PLANE('',#17088);
#15079=PLANE('',#17089);
#15080=PLANE('',#17091);
#15081=PLANE('',#17092);
#15082=PLANE('',#17093);
#15083=PLANE('',#17094);
#15084=PLANE('',#17095);
#15085=PLANE('',#17096);
#15694=ADVANCED_FACE('',(#2151),#15033,.T.);
#15695=ADVANCED_FACE('',(#2152),#15034,.T.);
#15696=ADVANCED_FACE('',(#2153),#15035,.T.);
#15697=ADVANCED_FACE('',(#2154),#15036,.T.);
#15698=ADVANCED_FACE('',(#2155),#15037,.T.);
#15699=ADVANCED_FACE('',(#2156),#15038,.T.);
#15700=ADVANCED_FACE('',(#2157),#15039,.T.);
#15701=ADVANCED_FACE('',(#2158),#15040,.T.);
#15702=ADVANCED_FACE('',(#2159),#501,.T.);
#15703=ADVANCED_FACE('',(#2160,#1188),#942,.T.);
#15704=ADVANCED_FACE('',(#2161),#943,.F.);
#15705=ADVANCED_FACE('',(#2162),#1746,.T.);
#15706=ADVANCED_FACE('',(#2163),#1747,.T.);
#15707=ADVANCED_FACE('',(#2164),#1748,.T.);
#15708=ADVANCED_FACE('',(#2165),#502,.T.);
#15709=ADVANCED_FACE('',(#2166,#1189),#944,.F.);
#15710=ADVANCED_FACE('',(#2167),#1749,.T.);
#15711=ADVANCED_FACE('',(#2168,#1190),#15041,.F.);
#15712=ADVANCED_FACE('',(#2169),#15042,.T.);
#15713=ADVANCED_FACE('',(#2170),#15043,.T.);
#15714=ADVANCED_FACE('',(#2171),#15044,.T.);
#15715=ADVANCED_FACE('',(#2172),#15045,.T.);
#15716=ADVANCED_FACE('',(#2173),#15046,.T.);
#15717=ADVANCED_FACE('',(#2174),#15047,.T.);
#15718=ADVANCED_FACE('',(#2175),#15048,.T.);
#15719=ADVANCED_FACE('',(#2176),#15049,.T.);
#15720=ADVANCED_FACE('',(#2177),#15050,.T.);
#15721=ADVANCED_FACE('',(#2178),#15051,.T.);
#15722=ADVANCED_FACE('',(#2179),#15052,.T.);
#15723=ADVANCED_FACE('',(#2180),#15053,.T.);
#15724=ADVANCED_FACE('',(#2181),#15054,.T.);
#15725=ADVANCED_FACE('',(#2182),#15055,.T.);
#15726=ADVANCED_FACE('',(#2183),#15056,.T.);
#15727=ADVANCED_FACE('',(#2184),#15057,.T.);
#15728=ADVANCED_FACE('',(#2185),#15058,.T.);
#15729=ADVANCED_FACE('',(#2186),#15059,.T.);
#15730=ADVANCED_FACE('',(#2187),#15060,.T.);
#15731=ADVANCED_FACE('',(#2188),#15061,.T.);
#15732=ADVANCED_FACE('',(#2189),#15062,.T.);
#15733=ADVANCED_FACE('',(#2190),#15063,.T.);
#15734=ADVANCED_FACE('',(#2191),#15064,.T.);
#15735=ADVANCED_FACE('',(#2192),#15065,.T.);
#15736=ADVANCED_FACE('',(#2193),#15066,.T.);
#15737=ADVANCED_FACE('',(#2194),#15067,.F.);
#15738=ADVANCED_FACE('',(#2195),#15068,.F.);
#15739=ADVANCED_FACE('',(#2196,#1191,#1192,#1193,#1194,#1195),#15069,.T.);
#15740=ADVANCED_FACE('',(#2197),#1750,.F.);
#15741=ADVANCED_FACE('',(#2198),#1751,.F.);
#15742=ADVANCED_FACE('',(#2199),#1752,.F.);
#15743=ADVANCED_FACE('',(#2200),#945,.F.);
#15744=ADVANCED_FACE('',(#2201),#1753,.F.);
#15745=ADVANCED_FACE('',(#2202),#946,.F.);
#15746=ADVANCED_FACE('',(#2203),#1754,.F.);
#15747=ADVANCED_FACE('',(#2204),#15070,.T.);
#15748=ADVANCED_FACE('',(#2205),#1755,.F.);
#15749=ADVANCED_FACE('',(#2206),#15071,.T.);
#15750=ADVANCED_FACE('',(#2207),#1756,.F.);
#15751=ADVANCED_FACE('',(#2208),#1757,.F.);
#15752=ADVANCED_FACE('',(#2209),#1758,.F.);
#15753=ADVANCED_FACE('',(#2210,#1196,#1197,#1198),#15072,.T.);
#15754=ADVANCED_FACE('',(#2211),#1759,.F.);
#15755=ADVANCED_FACE('',(#2212),#15073,.T.);
#15756=ADVANCED_FACE('',(#2213),#15074,.T.);
#15757=ADVANCED_FACE('',(#2214),#15075,.T.);
#15758=ADVANCED_FACE('',(#2215),#15076,.T.);
#15759=ADVANCED_FACE('',(#2216),#15077,.T.);
#15760=ADVANCED_FACE('',(#2217),#1760,.F.);
#15761=ADVANCED_FACE('',(#2218),#947,.F.);
#15762=ADVANCED_FACE('',(#2219),#1761,.F.);
#15763=ADVANCED_FACE('',(#2220),#1762,.F.);
#15764=ADVANCED_FACE('',(#2221),#1763,.F.);
#15765=ADVANCED_FACE('',(#2222),#15078,.F.);
#15766=ADVANCED_FACE('',(#2223),#15079,.T.);
#15767=ADVANCED_FACE('',(#2224),#1764,.F.);
#15768=ADVANCED_FACE('',(#2225),#15080,.F.);
#15769=ADVANCED_FACE('',(#2226),#15081,.T.);
#15770=ADVANCED_FACE('',(#2227),#15082,.T.);
#15771=ADVANCED_FACE('',(#2228),#15083,.T.);
#15772=ADVANCED_FACE('',(#2229),#15084,.T.);
#15773=ADVANCED_FACE('',(#2230),#15085,.T.);
#15774=ADVANCED_FACE('',(#2231),#948,.F.);
#16242=CLOSED_SHELL('',(#15694,#15695,#15696,#15697,#15698,#15699,#15700,
#15701,#15702,#15703,#15704,#15705,#15706,#15707,#15708,#15709,#15710,#15711,
#15712,#15713,#15714,#15715,#15716,#15717,#15718,#15719,#15720,#15721,#15722,
#15723,#15724,#15725,#15726,#15727,#15728,#15729,#15730,#15731,#15732,#15733,
#15734,#15735,#15736,#15737,#15738,#15739,#15740,#15741,#15742,#15743,#15744,
#15745,#15746,#15747,#15748,#15749,#15750,#15751,#15752,#15753,#15754,#15755,
#15756,#15757,#15758,#15759,#15760,#15761,#15762,#15763,#15764,#15765,#15766,
#15767,#15768,#15769,#15770,#15771,#15772,#15773,#15774));
#16983=AXIS2_PLACEMENT_3D('',#26834,#19522,#19523);
#16984=AXIS2_PLACEMENT_3D('',#26835,#19524,#19525);
#16985=AXIS2_PLACEMENT_3D('',#26848,#19532,#19533);
#16986=AXIS2_PLACEMENT_3D('',#26856,#19538,#19539);
#16987=AXIS2_PLACEMENT_3D('',#26862,#19543,#19544);
#16988=AXIS2_PLACEMENT_3D('',#26868,#19548,#19549);
#16989=AXIS2_PLACEMENT_3D('',#26877,#19554,#19555);
#16990=AXIS2_PLACEMENT_3D('',#26883,#19559,#19560);
#16991=AXIS2_PLACEMENT_3D('',#26889,#19564,#19565);
#16992=AXIS2_PLACEMENT_3D('',#26893,#19567,#19568);
#16993=AXIS2_PLACEMENT_3D('',#26895,#19569,#19570);
#16994=AXIS2_PLACEMENT_3D('',#27085,#19573,#19574);
#16995=AXIS2_PLACEMENT_3D('',#27087,#19575,#19576);
#16996=AXIS2_PLACEMENT_3D('',#27090,#19578,#19579);
#16997=AXIS2_PLACEMENT_3D('',#27092,#19580,#19581);
#16998=AXIS2_PLACEMENT_3D('',#27093,#19582,#19583);
#16999=AXIS2_PLACEMENT_3D('',#27094,#19584,#19585);
#17000=AXIS2_PLACEMENT_3D('',#27128,#19587,#19588);
#17001=AXIS2_PLACEMENT_3D('',#27134,#19589,#19590);
#17002=AXIS2_PLACEMENT_3D('',#27138,#19591,#19592);
#17003=AXIS2_PLACEMENT_3D('',#27140,#19593,#19594);
#17004=AXIS2_PLACEMENT_3D('',#27142,#19596,#19597);
#17005=AXIS2_PLACEMENT_3D('',#27144,#19598,#19599);
#17006=AXIS2_PLACEMENT_3D('',#27288,#19602,#19603);
#17007=AXIS2_PLACEMENT_3D('',#27290,#19604,#19605);
#17008=AXIS2_PLACEMENT_3D('',#27293,#19607,#19608);
#17009=AXIS2_PLACEMENT_3D('',#27294,#19609,#19610);
#17010=AXIS2_PLACEMENT_3D('',#27297,#19612,#19613);
#17011=AXIS2_PLACEMENT_3D('',#27298,#19614,#19615);
#17012=AXIS2_PLACEMENT_3D('',#27300,#19616,#19617);
#17013=AXIS2_PLACEMENT_3D('',#27301,#19618,#19619);
#17014=AXIS2_PLACEMENT_3D('',#27310,#19624,#19625);
#17015=AXIS2_PLACEMENT_3D('',#27316,#19629,#19630);
#17016=AXIS2_PLACEMENT_3D('',#27319,#19633,#19634);
#17017=AXIS2_PLACEMENT_3D('',#27322,#19637,#19638);
#17018=AXIS2_PLACEMENT_3D('',#27328,#19642,#19643);
#17019=AXIS2_PLACEMENT_3D('',#27329,#19644,#19645);
#17020=AXIS2_PLACEMENT_3D('',#27342,#19652,#19653);
#17021=AXIS2_PLACEMENT_3D('',#27352,#19659,#19660);
#17022=AXIS2_PLACEMENT_3D('',#27360,#19665,#19666);
#17023=AXIS2_PLACEMENT_3D('',#27364,#19669,#19670);
#17024=AXIS2_PLACEMENT_3D('',#27370,#19674,#19675);
#17025=AXIS2_PLACEMENT_3D('',#27379,#19681,#19682);
#17026=AXIS2_PLACEMENT_3D('',#27384,#19686,#19687);
#17027=AXIS2_PLACEMENT_3D('',#27386,#19689,#19690);
#17028=AXIS2_PLACEMENT_3D('',#27394,#19695,#19696);
#17029=AXIS2_PLACEMENT_3D('',#27398,#19699,#19700);
#17030=AXIS2_PLACEMENT_3D('',#27410,#19707,#19708);
#17031=AXIS2_PLACEMENT_3D('',#27414,#19710,#19711);
#17032=AXIS2_PLACEMENT_3D('',#27418,#19714,#19715);
#17033=AXIS2_PLACEMENT_3D('',#27422,#19718,#19719);
#17034=AXIS2_PLACEMENT_3D('',#27425,#19722,#19723);
#17035=AXIS2_PLACEMENT_3D('',#27431,#19727,#19728);
#17036=AXIS2_PLACEMENT_3D('',#27440,#19733,#19734);
#17037=AXIS2_PLACEMENT_3D('',#27449,#19739,#19740);
#17038=AXIS2_PLACEMENT_3D('',#27456,#19745,#19746);
#17039=AXIS2_PLACEMENT_3D('',#27463,#19751,#19752);
#17040=AXIS2_PLACEMENT_3D('',#27467,#19755,#19756);
#17041=AXIS2_PLACEMENT_3D('',#27471,#19759,#19760);
#17042=AXIS2_PLACEMENT_3D('',#27475,#19763,#19764);
#17043=AXIS2_PLACEMENT_3D('',#27477,#19765,#19766);
#17044=AXIS2_PLACEMENT_3D('',#27479,#19767,#19768);
#17045=AXIS2_PLACEMENT_3D('',#27481,#19769,#19770);
#17046=AXIS2_PLACEMENT_3D('',#27482,#19771,#19772);
#17047=AXIS2_PLACEMENT_3D('',#27485,#19774,#19775);
#17048=AXIS2_PLACEMENT_3D('',#27486,#19776,#19777);
#17049=AXIS2_PLACEMENT_3D('',#27489,#19779,#19780);
#17050=AXIS2_PLACEMENT_3D('',#27492,#19782,#19783);
#17051=AXIS2_PLACEMENT_3D('',#27493,#19784,#19785);
#17052=AXIS2_PLACEMENT_3D('',#27496,#19787,#19788);
#17053=AXIS2_PLACEMENT_3D('',#27497,#19789,#19790);
#17054=AXIS2_PLACEMENT_3D('',#27500,#19792,#19793);
#17055=AXIS2_PLACEMENT_3D('',#27501,#19794,#19795);
#17056=AXIS2_PLACEMENT_3D('',#27504,#19797,#19798);
#17057=AXIS2_PLACEMENT_3D('',#27505,#19799,#19800);
#17058=AXIS2_PLACEMENT_3D('',#27506,#19801,#19802);
#17059=AXIS2_PLACEMENT_3D('',#27507,#19803,#19804);
#17060=AXIS2_PLACEMENT_3D('',#27508,#19805,#19806);
#17061=AXIS2_PLACEMENT_3D('',#27509,#19807,#19808);
#17062=AXIS2_PLACEMENT_3D('',#27510,#19809,#19810);
#17063=AXIS2_PLACEMENT_3D('',#27511,#19811,#19812);
#17064=AXIS2_PLACEMENT_3D('',#27512,#19813,#19814);
#17065=AXIS2_PLACEMENT_3D('',#27514,#19815,#19816);
#17066=AXIS2_PLACEMENT_3D('',#27516,#19818,#19819);
#17067=AXIS2_PLACEMENT_3D('',#27519,#19821,#19822);
#17068=AXIS2_PLACEMENT_3D('',#27520,#19823,#19824);
#17069=AXIS2_PLACEMENT_3D('',#27522,#19825,#19826);
#17070=AXIS2_PLACEMENT_3D('',#27524,#19828,#19829);
#17071=AXIS2_PLACEMENT_3D('',#27534,#19834,#19835);
#17072=AXIS2_PLACEMENT_3D('',#27536,#19836,#19837);
#17073=AXIS2_PLACEMENT_3D('',#27537,#19838,#19839);
#17074=AXIS2_PLACEMENT_3D('',#27539,#19841,#19842);
#17075=AXIS2_PLACEMENT_3D('',#27543,#19846,#19847);
#17076=AXIS2_PLACEMENT_3D('',#27547,#19851,#19852);
#17077=AXIS2_PLACEMENT_3D('',#27548,#19853,#19854);
#17078=AXIS2_PLACEMENT_3D('',#27549,#19855,#19856);
#17079=AXIS2_PLACEMENT_3D('',#27552,#19859,#19860);
#17080=AXIS2_PLACEMENT_3D('',#27555,#19862,#19863);
#17081=AXIS2_PLACEMENT_3D('',#27556,#19864,#19865);
#17082=AXIS2_PLACEMENT_3D('',#27558,#19866,#19867);
#17083=AXIS2_PLACEMENT_3D('',#27560,#19869,#19870);
#17084=AXIS2_PLACEMENT_3D('',#27562,#19871,#19872);
#17085=AXIS2_PLACEMENT_3D('',#27564,#19874,#19875);
#17086=AXIS2_PLACEMENT_3D('',#27567,#19877,#19878);
#17087=AXIS2_PLACEMENT_3D('',#27568,#19879,#19880);
#17088=AXIS2_PLACEMENT_3D('',#27570,#19882,#19883);
#17089=AXIS2_PLACEMENT_3D('',#27572,#19885,#19886);
#17090=AXIS2_PLACEMENT_3D('',#27573,#19887,#19888);
#17091=AXIS2_PLACEMENT_3D('',#27575,#19890,#19891);
#17092=AXIS2_PLACEMENT_3D('',#27576,#19892,#19893);
#17093=AXIS2_PLACEMENT_3D('',#27577,#19894,#19895);
#17094=AXIS2_PLACEMENT_3D('',#27579,#19897,#19898);
#17095=AXIS2_PLACEMENT_3D('',#27580,#19899,#19900);
#17096=AXIS2_PLACEMENT_3D('',#27581,#19901,#19902);
#17097=AXIS2_PLACEMENT_3D('',#27583,#19904,#19905);
#19522=DIRECTION('axis',(0.,0.,1.));
#19523=DIRECTION('refdir',(1.,0.,0.));
#19524=DIRECTION('center_axis',(0.,-0.38268343236508,0.923879532511291));
#19525=DIRECTION('ref_axis',(1.,0.,0.));
#19526=DIRECTION('',(0.357406744336593,-0.86285620946102,-0.357406744336584));
#19527=DIRECTION('',(1.,0.,0.));
#19528=DIRECTION('',(0.357406744336593,0.86285620946102,0.357406744336584));
#19529=DIRECTION('',(-0.357406744336581,0.862856209461025,0.357406744336586));
#19530=DIRECTION('',(-1.,0.,0.));
#19531=DIRECTION('',(-0.357406744336581,-0.862856209461025,-0.357406744336586));
#19532=DIRECTION('center_axis',(0.707106781186553,0.,0.707106781186542));
#19533=DIRECTION('ref_axis',(0.707106781186542,0.,-0.707106781186553));
#19534=DIRECTION('',(-0.357406744336592,-0.862856209461016,0.357406744336597));
#19535=DIRECTION('',(0.,1.,0.));
#19536=DIRECTION('',(0.707106781186542,0.,-0.707106781186553));
#19537=DIRECTION('',(0.,-1.,0.));
#19538=DIRECTION('center_axis',(0.923879532511287,-0.382683432365088,0.));
#19539=DIRECTION('ref_axis',(0.,0.,-1.));
#19540=DIRECTION('',(0.,0.,-1.));
#19541=DIRECTION('',(0.281084637714813,0.678598344545841,0.678598344545856));
#19542=DIRECTION('',(0.,0.,1.));
#19543=DIRECTION('center_axis',(0.,-0.707106781186546,0.707106781186549));
#19544=DIRECTION('ref_axis',(1.,0.,0.));
#19545=DIRECTION('',(-0.577350269189625,0.577350269189627,0.577350269189625));
#19546=DIRECTION('',(-1.,0.,0.));
#19547=DIRECTION('',(-0.577350269189625,-0.577350269189627,-0.577350269189625));
#19548=DIRECTION('center_axis',(0.,-0.382683432365108,-0.923879532511279));
#19549=DIRECTION('ref_axis',(-1.,0.,0.));
#19550=DIRECTION('',(1.,0.,0.));
#19551=DIRECTION('',(0.678598344545848,-0.678598344545845,0.281084637714824));
#19552=DIRECTION('',(-1.,0.,0.));
#19553=DIRECTION('',(0.678598344545848,0.678598344545845,-0.281084637714824));
#19554=DIRECTION('center_axis',(0.382683432365094,0.,-0.923879532511285));
#19555=DIRECTION('ref_axis',(-0.923879532511285,0.,-0.382683432365094));
#19556=DIRECTION('',(0.,1.,0.));
#19557=DIRECTION('',(0.862856209461013,0.357406744336599,0.357406744336596));
#19558=DIRECTION('',(0.,-1.,0.));
#19559=DIRECTION('center_axis',(-0.382683432365094,0.,-0.923879532511285));
#19560=DIRECTION('ref_axis',(-0.923879532511285,0.,0.382683432365094));
#19561=DIRECTION('',(0.,1.,0.));
#19562=DIRECTION('',(0.862856209461013,-0.357406744336599,-0.357406744336596));
#19563=DIRECTION('',(0.,-1.,0.));
#19564=DIRECTION('center_axis',(0.,0.,-1.));
#19565=DIRECTION('ref_axis',(0.,1.,0.));
#19566=DIRECTION('',(-1.,0.,0.));
#19567=DIRECTION('center_axis',(0.,0.,1.));
#19568=DIRECTION('ref_axis',(1.,0.,0.));
#19569=DIRECTION('center_axis',(0.,0.,1.));
#19570=DIRECTION('ref_axis',(1.,0.,0.));
#19571=DIRECTION('',(-1.,0.,0.));
#19572=DIRECTION('',(-0.769134655216721,-0.639086756352105,0.));
#19573=DIRECTION('center_axis',(0.,0.,-1.));
#19574=DIRECTION('ref_axis',(1.,0.,0.));
#19575=DIRECTION('center_axis',(0.,0.,-1.));
#19576=DIRECTION('ref_axis',(1.,0.,0.));
#19577=DIRECTION('',(0.,0.,1.));
#19578=DIRECTION('center_axis',(0.,0.707106781186545,-0.70710678118655));
#19579=DIRECTION('ref_axis',(0.,-0.70710678118655,-0.707106781186545));
#19580=DIRECTION('center_axis',(0.,0.,1.));
#19581=DIRECTION('ref_axis',(1.,0.,0.));
#19582=DIRECTION('center_axis',(0.,0.707106781186545,-0.70710678118655));
#19583=DIRECTION('ref_axis',(0.,-0.70710678118655,-0.707106781186545));
#19584=DIRECTION('center_axis',(0.,1.,0.));
#19585=DIRECTION('ref_axis',(0.,0.,1.));
#19586=DIRECTION('',(0.,1.,0.));
#19587=DIRECTION('center_axis',(0.,0.,-1.));
#19588=DIRECTION('ref_axis',(1.,0.,0.));
#19589=DIRECTION('center_axis',(0.,0.,-1.));
#19590=DIRECTION('ref_axis',(1.,0.,0.));
#19591=DIRECTION('center_axis',(0.,-1.40939970598124E-15,1.));
#19592=DIRECTION('ref_axis',(1.,-3.03431454927927E-17,0.));
#19593=DIRECTION('center_axis',(0.,0.,1.));
#19594=DIRECTION('ref_axis',(1.,-6.12323399573677E-17,0.));
#19595=DIRECTION('',(-0.382683432365084,-1.2436385183643E-15,0.923879532511289));
#19596=DIRECTION('center_axis',(0.,0.,1.));
#19597=DIRECTION('ref_axis',(1.,0.,0.));
#19598=DIRECTION('center_axis',(0.,0.,-1.));
#19599=DIRECTION('ref_axis',(1.,-6.12323399573677E-17,0.));
#19600=DIRECTION('',(-0.707106781186549,8.65956056235495E-17,0.707106781186546));
#19601=DIRECTION('',(-0.123383141009019,0.711881246125774,-0.691376664293179));
#19602=DIRECTION('center_axis',(0.,0.,1.));
#19603=DIRECTION('ref_axis',(1.,0.,0.));
#19604=DIRECTION('center_axis',(0.,0.,1.));
#19605=DIRECTION('ref_axis',(1.,0.,0.));
#19606=DIRECTION('',(0.,0.,1.));
#19607=DIRECTION('center_axis',(0.,0.,1.));
#19608=DIRECTION('ref_axis',(1.,0.,0.));
#19609=DIRECTION('center_axis',(0.,3.38073055552685E-15,1.));
#19610=DIRECTION('ref_axis',(1.,-3.13005026890514E-17,0.));
#19611=DIRECTION('',(0.92387953251129,-1.20952485545349E-15,-0.382683432365083));
#19612=DIRECTION('center_axis',(0.,0.,1.));
#19613=DIRECTION('ref_axis',(1.,0.,0.));
#19614=DIRECTION('center_axis',(0.,0.,1.));
#19615=DIRECTION('ref_axis',(1.,0.,0.));
#19616=DIRECTION('center_axis',(0.,0.,-1.));
#19617=DIRECTION('ref_axis',(1.,0.,0.));
#19618=DIRECTION('center_axis',(0.,-0.923879532511289,-0.382683432365084));
#19619=DIRECTION('ref_axis',(0.,0.382683432365084,-0.923879532511289));
#19620=DIRECTION('',(1.,0.,0.));
#19621=DIRECTION('',(-0.678598344545838,-0.281084637714822,0.678598344545856));
#19622=DIRECTION('',(-1.,0.,0.));
#19623=DIRECTION('',(-0.678598344545838,0.281084637714822,-0.678598344545856));
#19624=DIRECTION('center_axis',(0.,-0.923879532511289,0.382683432365084));
#19625=DIRECTION('ref_axis',(0.,-0.382683432365084,-0.923879532511289));
#19626=DIRECTION('',(1.,0.,0.));
#19627=DIRECTION('',(0.678598344545835,0.28108463771482,0.678598344545859));
#19628=DIRECTION('',(0.678598344545835,-0.28108463771482,-0.678598344545859));
#19629=DIRECTION('center_axis',(0.382683432365093,-0.923879532511285,0.));
#19630=DIRECTION('ref_axis',(0.,0.,-1.));
#19631=DIRECTION('',(0.,0.,1.));
#19632=DIRECTION('',(0.,0.,-1.));
#19633=DIRECTION('center_axis',(-0.382683432365093,-0.923879532511285,0.));
#19634=DIRECTION('ref_axis',(0.,0.,-1.));
#19635=DIRECTION('',(0.,0.,-1.));
#19636=DIRECTION('',(0.,0.,1.));
#19637=DIRECTION('center_axis',(-0.707106781186549,-0.707106781186546,0.));
#19638=DIRECTION('ref_axis',(0.,0.,1.));
#19639=DIRECTION('',(0.,0.,1.));
#19640=DIRECTION('',(-0.577350269189625,0.577350269189628,0.577350269189625));
#19641=DIRECTION('',(0.577350269189624,-0.577350269189627,0.577350269189627));
#19642=DIRECTION('center_axis',(0.,-1.,0.));
#19643=DIRECTION('ref_axis',(0.,0.,-1.));
#19644=DIRECTION('center_axis',(0.707106781186542,0.,0.707106781186553));
#19645=DIRECTION('ref_axis',(0.707106781186553,0.,-0.707106781186542));
#19646=DIRECTION('',(0.577350269189628,0.577350269189631,-0.577350269189619));
#19647=DIRECTION('',(0.,1.,0.));
#19648=DIRECTION('',(-0.577350269189628,0.57735026918963,0.577350269189619));
#19649=DIRECTION('',(-0.577350269189634,-0.577350269189618,0.577350269189626));
#19650=DIRECTION('',(0.,-1.,0.));
#19651=DIRECTION('',(0.577350269189634,-0.577350269189617,-0.577350269189626));
#19652=DIRECTION('center_axis',(0.707106781186549,-0.707106781186546,0.));
#19653=DIRECTION('ref_axis',(0.,0.,-1.));
#19654=DIRECTION('',(-0.577350269189621,-0.577350269189624,-0.577350269189632));
#19655=DIRECTION('',(-0.357406744336593,-0.357406744336595,-0.862856209461016));
#19656=DIRECTION('',(0.,0.,-1.));
#19657=DIRECTION('',(0.707106781186546,0.707106781186549,0.));
#19658=DIRECTION('',(0.,0.,1.));
#19659=DIRECTION('center_axis',(0.,-0.707106781186553,0.707106781186542));
#19660=DIRECTION('ref_axis',(1.,0.,0.));
#19661=DIRECTION('',(-1.,0.,0.));
#19662=DIRECTION('',(0.577350269189634,0.577350269189617,0.577350269189626));
#19663=DIRECTION('',(-0.577350269189621,0.577350269189624,0.577350269189632));
#19664=DIRECTION('',(-1.,0.,0.));
#19665=DIRECTION('center_axis',(0.,0.,1.));
#19666=DIRECTION('ref_axis',(0.,-1.,0.));
#19667=DIRECTION('',(1.,0.,0.));
#19668=DIRECTION('',(0.,1.,0.));
#19669=DIRECTION('center_axis',(0.923879532511292,0.,-0.382683432365077));
#19670=DIRECTION('ref_axis',(-0.382683432365077,0.,-0.923879532511292));
#19671=DIRECTION('',(0.,1.,0.));
#19672=DIRECTION('',(0.357406744336583,-0.357406744336584,0.862856209461025));
#19673=DIRECTION('',(0.,-1.,0.));
#19674=DIRECTION('center_axis',(0.707106781186549,0.707106781186546,0.));
#19675=DIRECTION('ref_axis',(0.,0.,-1.));
#19676=DIRECTION('',(0.,0.,-1.));
#19677=DIRECTION('',(0.577350269189625,-0.577350269189628,0.577350269189625));
#19678=DIRECTION('',(-0.577350269189626,0.577350269189628,0.577350269189624));
#19679=DIRECTION('',(0.,0.,-1.));
#19680=DIRECTION('',(0.577350269189622,-0.577350269189624,0.577350269189632));
#19681=DIRECTION('center_axis',(0.707106781186548,0.,-0.707106781186548));
#19682=DIRECTION('ref_axis',(-0.707106781186548,0.,-0.707106781186548));
#19683=DIRECTION('',(0.577350269189625,0.577350269189628,0.577350269189625));
#19684=DIRECTION('',(-0.577350269189625,-0.577350269189628,-0.577350269189625));
#19685=DIRECTION('',(-0.577350269189626,0.577350269189626,-0.577350269189626));
#19686=DIRECTION('center_axis',(0.707106781186549,-0.707106781186546,0.));
#19687=DIRECTION('ref_axis',(0.,0.,-1.));
#19688=DIRECTION('',(0.577350269189624,0.577350269189627,-0.577350269189627));
#19689=DIRECTION('center_axis',(-0.923879532511292,0.,-0.382683432365077));
#19690=DIRECTION('ref_axis',(-0.382683432365077,0.,0.923879532511292));
#19691=DIRECTION('',(0.,1.,0.));
#19692=DIRECTION('',(0.357406744336583,0.357406744336584,-0.862856209461025));
#19693=DIRECTION('',(0.,-1.,0.));
#19694=DIRECTION('',(-0.281084637714813,0.678598344545841,0.678598344545856));
#19695=DIRECTION('center_axis',(-0.923879532511287,-0.382683432365088,0.));
#19696=DIRECTION('ref_axis',(0.,0.,1.));
#19697=DIRECTION('',(-0.357406744336592,0.862856209461016,-0.357406744336597));
#19698=DIRECTION('',(0.,0.,-1.));
#19699=DIRECTION('center_axis',(-0.707106781186549,0.707106781186546,0.));
#19700=DIRECTION('ref_axis',(0.,0.,1.));
#19701=DIRECTION('',(0.,0.,1.));
#19702=DIRECTION('',(-0.577350269189628,-0.57735026918963,-0.577350269189619));
#19703=DIRECTION('',(0.577350269189622,0.577350269189624,-0.577350269189632));
#19704=DIRECTION('',(0.,0.,1.));
#19705=DIRECTION('',(-0.577350269189626,-0.577350269189628,-0.577350269189624));
#19706=DIRECTION('',(0.577350269189625,0.577350269189628,-0.577350269189625));
#19707=DIRECTION('center_axis',(-1.,0.,0.));
#19708=DIRECTION('ref_axis',(0.,0.,1.));
#19709=DIRECTION('',(0.,-1.,0.));
#19710=DIRECTION('center_axis',(-1.,0.,0.));
#19711=DIRECTION('ref_axis',(0.,0.707106781186549,-0.707106781186546));
#19712=DIRECTION('',(0.,0.,-1.));
#19713=DIRECTION('',(0.,-1.,0.));
#19714=DIRECTION('center_axis',(-0.707106781186553,0.,0.707106781186542));
#19715=DIRECTION('ref_axis',(0.707106781186542,0.,0.707106781186553));
#19716=DIRECTION('',(0.,1.,0.));
#19717=DIRECTION('',(-0.707106781186542,0.,-0.707106781186553));
#19718=DIRECTION('center_axis',(-0.707106781186542,0.,0.707106781186553));
#19719=DIRECTION('ref_axis',(0.707106781186553,0.,0.707106781186542));
#19720=DIRECTION('',(0.577350269189628,-0.577350269189631,0.577350269189619));
#19721=DIRECTION('',(-0.577350269189634,0.577350269189618,-0.577350269189626));
#19722=DIRECTION('center_axis',(-0.707106781186549,-0.707106781186546,0.));
#19723=DIRECTION('ref_axis',(0.,0.,1.));
#19724=DIRECTION('',(-0.707106781186542,0.707106781186553,0.));
#19725=DIRECTION('',(0.,0.,1.));
#19726=DIRECTION('',(-0.357406744336593,0.357406744336595,0.862856209461016));
#19727=DIRECTION('center_axis',(-0.382683432365088,-0.923879532511288,0.));
#19728=DIRECTION('ref_axis',(0.,0.,-1.));
#19729=DIRECTION('',(0.,0.,1.));
#19730=DIRECTION('',(-0.862856209461024,0.357406744336595,-0.357406744336574));
#19731=DIRECTION('',(0.,0.,-1.));
#19732=DIRECTION('',(0.862856209461024,-0.357406744336595,-0.357406744336574));
#19733=DIRECTION('center_axis',(0.38268343236509,-0.923879532511287,0.));
#19734=DIRECTION('ref_axis',(0.,0.,-1.));
#19735=DIRECTION('',(0.,0.,-1.));
#19736=DIRECTION('',(0.862856209461024,0.357406744336597,0.357406744336571));
#19737=DIRECTION('',(0.,0.,1.));
#19738=DIRECTION('',(-0.862856209461024,-0.357406744336597,0.357406744336571));
#19739=DIRECTION('center_axis',(0.,-0.70710678118654,0.707106781186555));
#19740=DIRECTION('ref_axis',(1.,0.,0.));
#19741=DIRECTION('',(-1.,0.,0.));
#19742=DIRECTION('',(-0.57735026918963,-0.57735026918963,-0.577350269189618));
#19743=DIRECTION('',(1.,0.,0.));
#19744=DIRECTION('',(-0.57735026918963,0.57735026918963,0.577350269189618));
#19745=DIRECTION('center_axis',(0.,-0.70710678118654,-0.707106781186555));
#19746=DIRECTION('ref_axis',(-1.,0.,0.));
#19747=DIRECTION('',(-1.,0.,0.));
#19748=DIRECTION('',(0.57735026918963,0.57735026918963,-0.577350269189618));
#19749=DIRECTION('',(1.,0.,0.));
#19750=DIRECTION('',(0.57735026918963,-0.57735026918963,0.577350269189618));
#19751=DIRECTION('center_axis',(0.,0.,1.));
#19752=DIRECTION('ref_axis',(1.,0.,0.));
#19753=DIRECTION('',(-0.707106781186547,-0.707106781186548,0.));
#19754=DIRECTION('',(-0.707106781186547,0.707106781186548,0.));
#19755=DIRECTION('center_axis',(-0.707106781186548,0.707106781186547,0.));
#19756=DIRECTION('ref_axis',(-0.707106781186547,-0.707106781186548,0.));
#19757=DIRECTION('',(-0.707106781186547,-0.707106781186548,0.));
#19758=DIRECTION('',(0.,0.,1.));
#19759=DIRECTION('center_axis',(0.,-1.,0.));
#19760=DIRECTION('ref_axis',(0.,0.,-1.));
#19761=DIRECTION('',(-1.,0.,0.));
#19762=DIRECTION('',(1.,0.,0.));
#19763=DIRECTION('center_axis',(0.,-1.,0.));
#19764=DIRECTION('ref_axis',(1.,0.,0.));
#19765=DIRECTION('center_axis',(0.,-1.,0.));
#19766=DIRECTION('ref_axis',(0.,0.,1.));
#19767=DIRECTION('center_axis',(0.,-1.,0.));
#19768=DIRECTION('ref_axis',(1.,0.,0.));
#19769=DIRECTION('center_axis',(0.,-1.,0.));
#19770=DIRECTION('ref_axis',(0.,0.,1.));
#19771=DIRECTION('center_axis',(0.,-1.,0.));
#19772=DIRECTION('ref_axis',(1.,0.,0.));
#19773=DIRECTION('',(0.923879532511286,0.382683432365092,1.1314261122877E-16));
#19774=DIRECTION('center_axis',(0.,1.,0.));
#19775=DIRECTION('ref_axis',(1.,0.,0.));
#19776=DIRECTION('center_axis',(0.,-1.,0.));
#19777=DIRECTION('ref_axis',(1.,0.,0.));
#19778=DIRECTION('',(-0.707106781186547,-0.707106781186548,-8.65956056235493E-17));
#19779=DIRECTION('center_axis',(0.,-1.,0.));
#19780=DIRECTION('ref_axis',(0.,0.,1.));
#19781=DIRECTION('',(-8.65956056235497E-17,0.707106781186544,0.707106781186551));
#19782=DIRECTION('center_axis',(0.,1.,0.));
#19783=DIRECTION('ref_axis',(0.,0.,1.));
#19784=DIRECTION('center_axis',(0.,1.,0.));
#19785=DIRECTION('ref_axis',(0.,0.,1.));
#19786=DIRECTION('',(0.,1.,0.));
#19787=DIRECTION('center_axis',(0.,-1.,0.));
#19788=DIRECTION('ref_axis',(0.,0.,1.));
#19789=DIRECTION('center_axis',(0.,-1.,0.));
#19790=DIRECTION('ref_axis',(0.,0.,1.));
#19791=DIRECTION('',(-8.65956056235484E-17,0.707106781186555,0.70710678118654));
#19792=DIRECTION('center_axis',(0.,1.,0.));
#19793=DIRECTION('ref_axis',(0.,0.,1.));
#19794=DIRECTION('center_axis',(0.,1.,0.));
#19795=DIRECTION('ref_axis',(0.,0.,1.));
#19796=DIRECTION('',(0.,1.,0.));
#19797=DIRECTION('center_axis',(0.,-1.,0.));
#19798=DIRECTION('ref_axis',(0.,0.,1.));
#19799=DIRECTION('center_axis',(-1.,0.,0.));
#19800=DIRECTION('ref_axis',(0.,0.707106781186549,-0.707106781186546));
#19801=DIRECTION('center_axis',(1.,0.,0.));
#19802=DIRECTION('ref_axis',(0.,0.707106781186549,-0.707106781186546));
#19803=DIRECTION('center_axis',(0.,-0.923879532511286,0.382683432365092));
#19804=DIRECTION('ref_axis',(0.,-0.382683432365092,-0.923879532511286));
#19805=DIRECTION('center_axis',(1.,0.,0.));
#19806=DIRECTION('ref_axis',(0.,0.707106781186549,-0.707106781186546));
#19807=DIRECTION('center_axis',(-1.,0.,0.));
#19808=DIRECTION('ref_axis',(0.,0.707106781186549,-0.707106781186546));
#19809=DIRECTION('center_axis',(1.,0.,0.));
#19810=DIRECTION('ref_axis',(0.,0.707106781186549,-0.707106781186546));
#19811=DIRECTION('center_axis',(1.,0.,0.));
#19812=DIRECTION('ref_axis',(0.,0.,-1.));
#19813=DIRECTION('center_axis',(0.,-1.,0.));
#19814=DIRECTION('ref_axis',(1.,3.57124208663036E-17,0.));
#19815=DIRECTION('center_axis',(-7.26211808683936E-17,1.,-5.44658856512952E-17));
#19816=DIRECTION('ref_axis',(1.,7.26211808683936E-17,0.));
#19817=DIRECTION('',(-0.923879532511285,-0.382683432365094,1.1314261122877E-16));
#19818=DIRECTION('center_axis',(0.,-1.,0.));
#19819=DIRECTION('ref_axis',(1.,0.,0.));
#19820=DIRECTION('',(0.707106781186548,0.707106781186547,8.65956056235494E-17));
#19821=DIRECTION('center_axis',(7.29827365498645E-17,-1.,-2.00702525512128E-16));
#19822=DIRECTION('ref_axis',(1.,7.29827365498645E-17,0.));
#19823=DIRECTION('center_axis',(0.,1.,0.));
#19824=DIRECTION('ref_axis',(0.,0.,1.));
#19825=DIRECTION('center_axis',(0.,1.,0.));
#19826=DIRECTION('ref_axis',(0.,0.,1.));
#19827=DIRECTION('',(8.65956056235496E-17,-0.707106781186545,0.70710678118655));
#19828=DIRECTION('center_axis',(0.,1.,0.));
#19829=DIRECTION('ref_axis',(0.,0.,1.));
#19830=DIRECTION('',(1.,0.,0.));
#19831=DIRECTION('',(0.,0.,-1.));
#19832=DIRECTION('',(-1.,0.,0.));
#19833=DIRECTION('',(0.,0.,1.));
#19834=DIRECTION('center_axis',(0.,1.,0.));
#19835=DIRECTION('ref_axis',(0.,0.,1.));
#19836=DIRECTION('center_axis',(0.,1.,0.));
#19837=DIRECTION('ref_axis',(1.,0.,0.));
#19838=DIRECTION('center_axis',(0.,1.,0.));
#19839=DIRECTION('ref_axis',(0.,0.,1.));
#19840=DIRECTION('',(8.65956056235484E-17,-0.707106781186555,0.70710678118654));
#19841=DIRECTION('center_axis',(0.,0.923879532511296,0.382683432365068));
#19842=DIRECTION('ref_axis',(0.,-0.382683432365068,0.923879532511296));
#19843=DIRECTION('',(1.,0.,0.));
#19844=DIRECTION('',(-0.678598344545828,0.281084637714811,-0.67859834454587));
#19845=DIRECTION('',(-0.678598344545828,-0.281084637714811,0.67859834454587));
#19846=DIRECTION('center_axis',(0.,0.923879532511288,-0.382683432365088));
#19847=DIRECTION('ref_axis',(0.,0.382683432365088,0.923879532511288));
#19848=DIRECTION('',(0.678598344545841,-0.281084637714821,-0.678598344545853));
#19849=DIRECTION('',(-1.,0.,0.));
#19850=DIRECTION('',(0.678598344545841,0.281084637714821,0.678598344545853));
#19851=DIRECTION('center_axis',(0.382683432365095,0.923879532511285,0.));
#19852=DIRECTION('ref_axis',(0.,0.,1.));
#19853=DIRECTION('center_axis',(-0.382683432365095,0.923879532511285,0.));
#19854=DIRECTION('ref_axis',(0.,0.,1.));
#19855=DIRECTION('center_axis',(0.,0.707106781186545,-0.70710678118655));
#19856=DIRECTION('ref_axis',(-1.,0.,0.));
#19857=DIRECTION('',(-1.,0.,0.));
#19858=DIRECTION('',(0.577350269189625,-0.577350269189628,-0.577350269189625));
#19859=DIRECTION('center_axis',(0.,-1.,0.));
#19860=DIRECTION('ref_axis',(1.,3.67475894571974E-17,0.));
#19861=DIRECTION('',(0.38268343236509,0.923879532511286,4.68652040532631E-17));
#19862=DIRECTION('center_axis',(0.,1.,0.));
#19863=DIRECTION('ref_axis',(1.,0.,0.));
#19864=DIRECTION('center_axis',(0.,-1.,0.));
#19865=DIRECTION('ref_axis',(1.,0.,0.));
#19866=DIRECTION('center_axis',(0.,-1.,0.));
#19867=DIRECTION('ref_axis',(1.,0.,0.));
#19868=DIRECTION('',(0.,-1.,0.));
#19869=DIRECTION('center_axis',(-5.23364152894587E-15,1.,0.));
#19870=DIRECTION('ref_axis',(1.,0.,0.));
#19871=DIRECTION('center_axis',(0.,-1.,-7.26211808683936E-17));
#19872=DIRECTION('ref_axis',(1.,0.,0.));
#19873=DIRECTION('',(-0.923879532511287,0.38268343236509,-1.1314261122877E-16));
#19874=DIRECTION('center_axis',(0.,1.,0.));
#19875=DIRECTION('ref_axis',(1.,0.,0.));
#19876=DIRECTION('',(0.707106781186547,-0.707106781186547,-8.65956056235493E-17));
#19877=DIRECTION('center_axis',(0.,1.,1.45965473099729E-16));
#19878=DIRECTION('ref_axis',(1.,0.,0.));
#19879=DIRECTION('center_axis',(2.16784530188845E-15,1.,0.));
#19880=DIRECTION('ref_axis',(1.,0.,0.));
#19881=DIRECTION('',(0.382683432365085,-0.923879532511289,-4.68652040532626E-17));
#19882=DIRECTION('center_axis',(0.707106781186548,0.707106781186547,0.));
#19883=DIRECTION('ref_axis',(-0.707106781186547,0.707106781186548,0.));
#19884=DIRECTION('',(-0.707106781186547,0.707106781186548,0.));
#19885=DIRECTION('center_axis',(0.,0.,1.));
#19886=DIRECTION('ref_axis',(1.,0.,0.));
#19887=DIRECTION('center_axis',(0.,0.,-1.));
#19888=DIRECTION('ref_axis',(1.,0.,0.));
#19889=DIRECTION('',(0.707106781186547,-8.65956056235493E-17,0.707106781186547));
#19890=DIRECTION('center_axis',(0.,0.,1.));
#19891=DIRECTION('ref_axis',(1.,0.,0.));
#19892=DIRECTION('center_axis',(0.,0.,1.));
#19893=DIRECTION('ref_axis',(1.,0.,0.));
#19894=DIRECTION('center_axis',(0.,-0.707106781186548,-0.707106781186548));
#19895=DIRECTION('ref_axis',(-1.,0.,0.));
#19896=DIRECTION('',(-0.577350269189626,-0.577350269189626,0.577350269189626));
#19897=DIRECTION('center_axis',(-0.707106781186548,0.,-0.707106781186548));
#19898=DIRECTION('ref_axis',(-0.707106781186548,0.,0.707106781186548));
#19899=DIRECTION('center_axis',(0.,0.707106781186552,0.707106781186543));
#19900=DIRECTION('ref_axis',(1.,0.,0.));
#19901=DIRECTION('center_axis',(0.,0.,1.));
#19902=DIRECTION('ref_axis',(0.,-1.,0.));
#19903=DIRECTION('',(1.,0.,0.));
#19904=DIRECTION('center_axis',(1.,0.,0.));
#19905=DIRECTION('ref_axis',(0.,0.707106781186549,-0.707106781186546));
#26834=CARTESIAN_POINT('',(0.,0.,0.));
#26835=CARTESIAN_POINT('Origin',(0.,-1.3456066017178,6.2893933982822));
#26836=CARTESIAN_POINT('',(-2.885,-1.3562132034356,6.285));
#26837=CARTESIAN_POINT('',(-2.8787867965644,-1.3712132034356,6.2787867965644));
#26838=CARTESIAN_POINT('',(-2.82767686307234,-1.49460349804412,6.22767686307234));
#26839=CARTESIAN_POINT('',(2.8787867965644,-1.3712132034356,6.2787867965644));
#26840=CARTESIAN_POINT('',(0.,-1.3712132034356,6.2787867965644));
#26841=CARTESIAN_POINT('',(2.885,-1.3562132034356,6.285));
#26842=CARTESIAN_POINT('',(2.82767686307234,-1.49460349804412,6.22767686307234));
#26843=CARTESIAN_POINT('',(2.87,-1.32,6.3));
#26844=CARTESIAN_POINT('',(2.489697839644,-0.401869366668709,6.68030216035601));
#26845=CARTESIAN_POINT('',(-2.87,-1.32,6.3));
#26846=CARTESIAN_POINT('',(0.,-1.32,6.3));
#26847=CARTESIAN_POINT('',(-2.489697839644,-0.401869366668709,6.68030216035601));
#26848=CARTESIAN_POINT('Origin',(2.885,2.77555756156289E-17,6.285));
#26849=CARTESIAN_POINT('',(2.9,-1.32,6.27));
#26850=CARTESIAN_POINT('',(2.97292879382193,-1.14393431686758,6.19707120617807));
#26851=CARTESIAN_POINT('',(2.9,0.1,6.27));
#26852=CARTESIAN_POINT('',(2.9,2.77555756156289E-17,6.27));
#26853=CARTESIAN_POINT('',(2.87,0.1,6.3));
#26854=CARTESIAN_POINT('',(2.87,0.1,6.3));
#26855=CARTESIAN_POINT('',(2.87,2.77555756156289E-17,6.3));
#26856=CARTESIAN_POINT('Origin',(2.8893933982822,-1.3456066017178,8.2125));
#26857=CARTESIAN_POINT('',(2.8787867965644,-1.3712132034356,5.7287867965644));
#26858=CARTESIAN_POINT('',(2.8787867965644,-1.3712132034356,8.2125));
#26859=CARTESIAN_POINT('',(2.9,-1.32,5.78));
#26860=CARTESIAN_POINT('',(2.8787867965644,-1.3712132034356,5.7287867965644));
#26861=CARTESIAN_POINT('',(2.9,-1.32,8.2125));
#26862=CARTESIAN_POINT('Origin',(0.,-1.375,6.275));
#26863=CARTESIAN_POINT('',(-2.8712132034356,-1.3787867965644,6.2712132034356));
#26864=CARTESIAN_POINT('',(-2.6125,-1.6375,6.0125));
#26865=CARTESIAN_POINT('',(2.8712132034356,-1.3787867965644,6.2712132034356));
#26866=CARTESIAN_POINT('',(0.,-1.3787867965644,6.2712132034356));
#26867=CARTESIAN_POINT('',(2.6125,-1.6375,6.0125));
#26868=CARTESIAN_POINT('Origin',(0.,-1.3456066017178,5.7106066017178));
#26869=CARTESIAN_POINT('',(-2.82,-1.32,5.7));
#26870=CARTESIAN_POINT('',(2.82,-1.32,5.7));
#26871=CARTESIAN_POINT('',(0.,-1.32,5.7));
#26872=CARTESIAN_POINT('',(2.8712132034356,-1.3712132034356,5.7212132034356));
#26873=CARTESIAN_POINT('',(2.82,-1.32,5.7));
#26874=CARTESIAN_POINT('',(-2.8712132034356,-1.3712132034356,5.7212132034356));
#26875=CARTESIAN_POINT('',(0.,-1.3712132034356,5.7212132034356));
#26876=CARTESIAN_POINT('',(-2.8712132034356,-1.3712132034356,5.7212132034356));
#26877=CARTESIAN_POINT('Origin',(2.8456066017178,-1.1,5.7106066017178));
#26878=CARTESIAN_POINT('',(2.82,0.95,5.7));
#26879=CARTESIAN_POINT('',(2.82,-1.1,5.7));
#26880=CARTESIAN_POINT('',(2.8712132034356,0.971213203435597,5.7212132034356));
#26881=CARTESIAN_POINT('',(1.47300280204935,0.392055492130272,5.14205549213028));
#26882=CARTESIAN_POINT('',(2.8712132034356,-1.1,5.7212132034356));
#26883=CARTESIAN_POINT('Origin',(-2.8456066017178,-1.1,5.7106066017178));
#26884=CARTESIAN_POINT('',(-2.8712132034356,0.971213203435597,5.7212132034356));
#26885=CARTESIAN_POINT('',(-2.8712132034356,-1.1,5.7212132034356));
#26886=CARTESIAN_POINT('',(-2.82,0.95,5.7));
#26887=CARTESIAN_POINT('',(-1.47300280204935,0.392055492130272,5.14205549213028));
#26888=CARTESIAN_POINT('',(-2.82,-1.1,5.7));
#26889=CARTESIAN_POINT('Origin',(0.,-1.4,5.7));
#26890=CARTESIAN_POINT('',(-0.733143914930758,0.950000000000001,5.7));
#26891=CARTESIAN_POINT('',(0.,0.95,5.7));
#26892=CARTESIAN_POINT('',(-1.2,1.46957615897682E-16,5.7));
#26893=CARTESIAN_POINT('Origin',(0.,0.,5.7));
#26894=CARTESIAN_POINT('',(0.733143914930758,0.950000000000001,5.7));
#26895=CARTESIAN_POINT('Origin',(0.,0.,5.7));
#26896=CARTESIAN_POINT('',(0.,0.95,5.7));
#26897=CARTESIAN_POINT('Ctrl Pts',(0.234492626320026,1.17686584120771,5.2));
#26898=CARTESIAN_POINT('Ctrl Pts',(0.234492626320026,1.17686584120771,5.21851592037048));
#26899=CARTESIAN_POINT('Ctrl Pts',(0.230065594000457,1.17776475629821,5.25703220095455));
#26900=CARTESIAN_POINT('Ctrl Pts',(0.208561308949327,1.18184858998349,5.31286098873592));
#26901=CARTESIAN_POINT('Ctrl Pts',(0.175078618630889,1.18735985109294,5.35981780168936));
#26902=CARTESIAN_POINT('Ctrl Pts',(0.132977608595357,1.19291479882069,5.39638849063154));
#26903=CARTESIAN_POINT('Ctrl Pts',(0.0797919333124946,1.19779759041496,
5.42375237476982));
#26904=CARTESIAN_POINT('Ctrl Pts',(0.0270809220838994,1.20001767329007,
5.43500694450787));
#26905=CARTESIAN_POINT('Ctrl Pts',(-0.0286029864222697,1.20010475087302,
5.43548184690207));
#26906=CARTESIAN_POINT('Ctrl Pts',(-0.0673004953048968,1.19832870594691,
5.42640311279717));
#26907=CARTESIAN_POINT('Ctrl Pts',(-0.118808426842686,1.19445759764994,
5.40509087371658));
#26908=CARTESIAN_POINT('Ctrl Pts',(-0.145105499862307,1.19138154283581,
5.38703853259485));
#26909=CARTESIAN_POINT('Ctrl Pts',(-0.186607973526257,1.18557851967241,
5.34540463031795));
#26910=CARTESIAN_POINT('Ctrl Pts',(-0.204599918973935,1.18248717481483,
5.31905282963216));
#26911=CARTESIAN_POINT('Ctrl Pts',(-0.228496361591337,1.17808596546445,
5.26111603578263));
#26912=CARTESIAN_POINT('Ctrl Pts',(-0.234425323120645,1.17685953455129,
5.22956894464554));
#26913=CARTESIAN_POINT('Ctrl Pts',(-0.234294478758728,1.17688759738335,
5.17767894605582));
#26914=CARTESIAN_POINT('Ctrl Pts',(-0.228111094333853,1.17818452128479,
5.13119983678783));
#26915=CARTESIAN_POINT('Ctrl Pts',(-0.196601450552936,1.18397925051513,
5.06597720676137));
#26916=CARTESIAN_POINT('Ctrl Pts',(-0.152167749680949,1.19070622188097,
5.01676689334197));
#26917=CARTESIAN_POINT('Ctrl Pts',(-0.0915400219194833,1.19713526569684,
4.97952753552852));
#26918=CARTESIAN_POINT('Ctrl Pts',(-0.0222401922789184,1.20045910805244,
4.96273883536335));
#26919=CARTESIAN_POINT('Ctrl Pts',(0.0335828950866025,1.19987839029729,
4.96556047978417));
#26920=CARTESIAN_POINT('Ctrl Pts',(0.102259384899266,1.19636361322958,4.98396469296537));
#26921=CARTESIAN_POINT('Ctrl Pts',(0.142497929826391,1.19174220944178,5.01030250445097));
#26922=CARTESIAN_POINT('Ctrl Pts',(0.186690885906675,1.18557585757076,5.05453934674594));
#26923=CARTESIAN_POINT('Ctrl Pts',(0.204662083875366,1.18248576762501,5.08088946271256));
#26924=CARTESIAN_POINT('Ctrl Pts',(0.228592229859133,1.1780835276557,5.13881431659721));
#26925=CARTESIAN_POINT('Ctrl Pts',(0.234492626320026,1.17686584120771,5.17037400265145));
#26926=CARTESIAN_POINT('Ctrl Pts',(0.234492626320026,1.17686584120771,5.2));
#26927=CARTESIAN_POINT('Ctrl Pts',(0.224661750880017,1.16869720356482,5.2));
#26928=CARTESIAN_POINT('Ctrl Pts',(0.224664044082871,1.16869658022503,5.21784968514182));
#26929=CARTESIAN_POINT('Ctrl Pts',(0.220347781825578,1.16953151025151,5.25499826456546));
#26930=CARTESIAN_POINT('Ctrl Pts',(0.199462940996693,1.17331171992303,5.30869422291513));
#26931=CARTESIAN_POINT('Ctrl Pts',(0.167106453640583,1.17839956757166,5.35364934929127));
#26932=CARTESIAN_POINT('Ctrl Pts',(0.126660674993384,1.1835094683978,5.38846950726549));
#26933=CARTESIAN_POINT('Ctrl Pts',(0.0758545072020466,1.18798593044828,
5.41438801389221));
#26934=CARTESIAN_POINT('Ctrl Pts',(0.0257341972508752,1.19001518718189,
5.42499940578561));
#26935=CARTESIAN_POINT('Ctrl Pts',(-0.0271662575703232,1.19009521901816,
5.4254491044883));
#26936=CARTESIAN_POINT('Ctrl Pts',(-0.0639694888884449,1.18847148693327,
5.41688611040433));
#26937=CARTESIAN_POINT('Ctrl Pts',(-0.113097318603888,1.18492738150962,
5.39672394786756));
#26938=CARTESIAN_POINT('Ctrl Pts',(-0.138291037166866,1.1821013903319,5.37958710544409));
#26939=CARTESIAN_POINT('Ctrl Pts',(-0.178227153593058,1.17675766202459,
5.33986702046425));
#26940=CARTESIAN_POINT('Ctrl Pts',(-0.195628209030011,1.17390150521058,
5.31462522547444));
#26941=CARTESIAN_POINT('Ctrl Pts',(-0.218819386947306,1.16982933241391,
5.25892872162705));
#26942=CARTESIAN_POINT('Ctrl Pts',(-0.224587941395262,1.1686929086115,5.2285063395467));
#26943=CARTESIAN_POINT('Ctrl Pts',(-0.224471866771419,1.1687172800089,5.17847879299728));
#26944=CARTESIAN_POINT('Ctrl Pts',(-0.218433291914077,1.16992270346931,
5.13365077066068));
#26945=CARTESIAN_POINT('Ctrl Pts',(-0.187868345911638,1.17528340489058,
5.07099553678837));
#26946=CARTESIAN_POINT('Ctrl Pts',(-0.145053403930571,1.18148068253972,
5.02402161588194));
#26947=CARTESIAN_POINT('Ctrl Pts',(-0.0870347413400359,1.18738127001952,
4.98869879876734));
#26948=CARTESIAN_POINT('Ctrl Pts',(-0.0211261762958701,1.19041889729488,
4.97287241139659));
#26949=CARTESIAN_POINT('Ctrl Pts',(0.0318967819082349,1.18988874316386,
4.97552771036542));
#26950=CARTESIAN_POINT('Ctrl Pts',(0.0972569740091445,1.18667356122128,
4.9929056676729));
#26951=CARTESIAN_POINT('Ctrl Pts',(0.135784681753249,1.18243415718769,5.01787150746554));
#26952=CARTESIAN_POINT('Ctrl Pts',(0.178307565473129,1.17675446720244,5.06007864635613));
#26953=CARTESIAN_POINT('Ctrl Pts',(0.195692635440334,1.1739004547617,5.08531514197247));
#26954=CARTESIAN_POINT('Ctrl Pts',(0.218912554144602,1.16982655564952,5.14100422188478));
#26955=CARTESIAN_POINT('Ctrl Pts',(0.224660105409413,1.16869963356623,5.17143164799448));
#26956=CARTESIAN_POINT('Ctrl Pts',(0.224661750880017,1.16869720356482,5.2));
#26957=CARTESIAN_POINT('Ctrl Pts',(0.214830875440008,1.16052856592193,5.2));
#26958=CARTESIAN_POINT('Ctrl Pts',(0.214828582237154,1.16052918926171,5.21719693319092));
#26959=CARTESIAN_POINT('Ctrl Pts',(0.210634710406464,1.16129601125582,5.25295676722098));
#26960=CARTESIAN_POINT('Ctrl Pts',(0.190362570396196,1.16477491560071,5.30453079295661));
#26961=CARTESIAN_POINT('Ctrl Pts',(0.159134503245928,1.16944043352991,5.34748758598507));
#26962=CARTESIAN_POINT('Ctrl Pts',(0.120331596908531,1.17410858214668,5.38057170621492));
#26963=CARTESIAN_POINT('Ctrl Pts',(0.0719132086075718,1.17817752530137,
5.40503842533525));
#26964=CARTESIAN_POINT('Ctrl Pts',(0.0243663461721618,1.18001467471676,
5.4150055273476));
#26965=CARTESIAN_POINT('Ctrl Pts',(-0.0257415711068092,1.18008692449041,
5.41542929395432));
#26966=CARTESIAN_POINT('Ctrl Pts',(-0.0606502732383226,1.1786161400379,
5.40738216145846));
#26967=CARTESIAN_POINT('Ctrl Pts',(-0.107389914733047,1.17539276698966,
5.38835446764134));
#26968=CARTESIAN_POINT('Ctrl Pts',(-0.131489864383231,1.17282131064298,
5.3721457714085));
#26969=CARTESIAN_POINT('Ctrl Pts',(-0.169849523031342,1.16793341659147,
5.33433090190193));
#26970=CARTESIAN_POINT('Ctrl Pts',(-0.186680035883757,1.16531442344864,
5.31021018521442));
#26971=CARTESIAN_POINT('Ctrl Pts',(-0.209144973553841,1.16157006705547,
5.2567474710098));
#26972=CARTESIAN_POINT('Ctrl Pts',(-0.214785043930596,1.16052068738504,
5.22746776581041));
#26973=CARTESIAN_POINT('Ctrl Pts',(-0.214649541396742,1.16054630709438,
5.17927946000339));
#26974=CARTESIAN_POINT('Ctrl Pts',(-0.208777651148686,1.16165383773602,
5.13611567681124));
#26975=CARTESIAN_POINT('Ctrl Pts',(-0.179153953237642,1.16658250125997,
5.0760273252867));
#26976=CARTESIAN_POINT('Ctrl Pts',(-0.137910376824399,1.17226130085929,
5.03125163794571));
#26977=CARTESIAN_POINT('Ctrl Pts',(-0.0825171178287952,1.17762891532049,
4.99786508496316));
#26978=CARTESIAN_POINT('Ctrl Pts',(-0.0199848479662072,1.18038001208676,
4.98300022887185));
#26979=CARTESIAN_POINT('Ctrl Pts',(0.0302169894530887,1.17989998331047,
4.98549037212516));
#26980=CARTESIAN_POINT('Ctrl Pts',(0.0922643071693305,1.17698583602376,
5.00183735778633));
#26981=CARTESIAN_POINT('Ctrl Pts',(0.129073305025927,1.17312581435099,5.02543896237632));
#26982=CARTESIAN_POINT('Ctrl Pts',(0.169922090789214,1.167932896833,5.06561751781489));
#26983=CARTESIAN_POINT('Ctrl Pts',(0.186728468423531,1.16531399806998,5.08974201762226));
#26984=CARTESIAN_POINT('Ctrl Pts',(0.209226990165204,1.16156954658368,5.14319234394881));
#26985=CARTESIAN_POINT('Ctrl Pts',(0.214832520910613,1.16052613592052,5.17249276942433));
#26986=CARTESIAN_POINT('Ctrl Pts',(0.214830875440008,1.16052856592193,5.2));
#26987=CARTESIAN_POINT('Ctrl Pts',(0.204999999999999,1.15235992827903,5.2));
#26988=CARTESIAN_POINT('Ctrl Pts',(0.204999999999999,1.15235992827903,5.21653069796226));
#26989=CARTESIAN_POINT('Ctrl Pts',(0.200916898231585,1.15306276520912,5.25092283083188));
#26990=CARTESIAN_POINT('Ctrl Pts',(0.181264202443562,1.15623804554025,5.30036402713581));
#26991=CARTESIAN_POINT('Ctrl Pts',(0.151162338255622,1.16048015000863,5.34131913358699));
#26992=CARTESIAN_POINT('Ctrl Pts',(0.114014663306557,1.16470325172378,5.37265272284888));
#26993=CARTESIAN_POINT('Ctrl Pts',(0.0679757824971238,1.16836586533469,
5.39567406445764));
#26994=CARTESIAN_POINT('Ctrl Pts',(0.0230196213391375,1.17001218860859,
5.40499798862534));
#26995=CARTESIAN_POINT('Ctrl Pts',(-0.0243048422548627,1.17007739263555,
5.40539655154055));
#26996=CARTESIAN_POINT('Ctrl Pts',(-0.0573192668218707,1.16875892102426,
5.39786515906562));
#26997=CARTESIAN_POINT('Ctrl Pts',(-0.101678806494249,1.16586255084935,
5.37998754179231));
#26998=CARTESIAN_POINT('Ctrl Pts',(-0.124675401687789,1.16354115813907,
5.36469434425773));
#26999=CARTESIAN_POINT('Ctrl Pts',(-0.161468703098142,1.15911255894365,
5.32879329204822));
#27000=CARTESIAN_POINT('Ctrl Pts',(-0.177708325939833,1.15672875384439,
5.30578258105671));
#27001=CARTESIAN_POINT('Ctrl Pts',(-0.19946799890981,1.15331343400492,5.25456015685422));
#27002=CARTESIAN_POINT('Ctrl Pts',(-0.204947662205213,1.15235406144525,
5.22640516071157));
#27003=CARTESIAN_POINT('Ctrl Pts',(-0.204826929409432,1.15237598971992,
5.18007930694485));
#27004=CARTESIAN_POINT('Ctrl Pts',(-0.19909984872891,1.15339201992053,5.13856661068409));
#27005=CARTESIAN_POINT('Ctrl Pts',(-0.170420848596344,1.15788665563542,
5.08104565531369));
#27006=CARTESIAN_POINT('Ctrl Pts',(-0.130796031074021,1.16303576151804,
5.03850636048567));
#27007=CARTESIAN_POINT('Ctrl Pts',(-0.0780118372493478,1.16787491964318,
5.00703634820198));
#27008=CARTESIAN_POINT('Ctrl Pts',(-0.0188708319831588,1.1703398013292,
4.99313380490508));
#27009=CARTESIAN_POINT('Ctrl Pts',(0.0285308762747211,1.16991033617703,
4.99545760270642));
#27010=CARTESIAN_POINT('Ctrl Pts',(0.0872618962792086,1.16729578401546,
5.01077833249387));
#27011=CARTESIAN_POINT('Ctrl Pts',(0.122360056952786,1.16381776209691,5.03300796539089));
#27012=CARTESIAN_POINT('Ctrl Pts',(0.161538770355668,1.15911150646468,5.07115681742508));
#27013=CARTESIAN_POINT('Ctrl Pts',(0.177759019988499,1.15672868520667,5.09416769688216));
#27014=CARTESIAN_POINT('Ctrl Pts',(0.199547314450672,1.1533125745775,5.14538224923639));
#27015=CARTESIAN_POINT('Ctrl Pts',(0.204999999999999,1.15235992827903,5.17355041476736));
#27016=CARTESIAN_POINT('Ctrl Pts',(0.204999999999999,1.15235992827903,5.2));
#27017=CARTESIAN_POINT('',(0.234492626320026,1.17686584120771,5.2));
#27018=CARTESIAN_POINT('',(0.204999999999999,1.15235992827903,5.2));
#27019=CARTESIAN_POINT('',(0.234492626320026,1.17686584120771,5.2));
#27020=CARTESIAN_POINT('',(-4.97473164011138E-6,1.17000356538632,4.99499072157072));
#27021=CARTESIAN_POINT('Ctrl Pts',(0.204999999999999,1.15235992827903,5.2));
#27022=CARTESIAN_POINT('Ctrl Pts',(0.204999999999999,1.15235992827903,5.21653069796226));
#27023=CARTESIAN_POINT('Ctrl Pts',(0.200916898231585,1.15306276520912,5.25092283083188));
#27024=CARTESIAN_POINT('Ctrl Pts',(0.181264202443562,1.15623804554025,5.30036402713581));
#27025=CARTESIAN_POINT('Ctrl Pts',(0.151162338255622,1.16048015000863,5.34131913358699));
#27026=CARTESIAN_POINT('Ctrl Pts',(0.114014663306557,1.16470325172378,5.37265272284888));
#27027=CARTESIAN_POINT('Ctrl Pts',(0.0679757824971238,1.16836586533469,
5.39567406445764));
#27028=CARTESIAN_POINT('Ctrl Pts',(0.0230196213391375,1.17001218860859,
5.40499798862534));
#27029=CARTESIAN_POINT('Ctrl Pts',(-0.0243048422548627,1.17007739263555,
5.40539655154055));
#27030=CARTESIAN_POINT('Ctrl Pts',(-0.0573192668218707,1.16875892102426,
5.39786515906562));
#27031=CARTESIAN_POINT('Ctrl Pts',(-0.101678806494249,1.16586255084935,
5.37998754179231));
#27032=CARTESIAN_POINT('Ctrl Pts',(-0.124675401687789,1.16354115813907,
5.36469434425773));
#27033=CARTESIAN_POINT('Ctrl Pts',(-0.161468703098142,1.15911255894365,
5.32879329204822));
#27034=CARTESIAN_POINT('Ctrl Pts',(-0.177708325939833,1.15672875384439,
5.30578258105671));
#27035=CARTESIAN_POINT('Ctrl Pts',(-0.19946799890981,1.15331343400492,5.25456015685422));
#27036=CARTESIAN_POINT('Ctrl Pts',(-0.204947662205213,1.15235406144525,
5.22640516071157));
#27037=CARTESIAN_POINT('Ctrl Pts',(-0.204826929409432,1.15237598971992,
5.18007930694485));
#27038=CARTESIAN_POINT('Ctrl Pts',(-0.19909984872891,1.15339201992053,5.13856661068409));
#27039=CARTESIAN_POINT('Ctrl Pts',(-0.170420848596344,1.15788665563542,
5.08104565531369));
#27040=CARTESIAN_POINT('Ctrl Pts',(-0.130796031074021,1.16303576151804,
5.03850636048567));
#27041=CARTESIAN_POINT('Ctrl Pts',(-0.0780118372493478,1.16787491964318,
5.00703634820198));
#27042=CARTESIAN_POINT('Ctrl Pts',(-0.032012760281176,1.16979207140417,
4.99622313736308));
#27043=CARTESIAN_POINT('Ctrl Pts',(-0.00639669818699399,1.17000452714276,
4.99498981359792));
#27044=CARTESIAN_POINT('Ctrl Pts',(-4.97473164011615E-6,1.17000356538632,
4.99499072157072));
#27045=CARTESIAN_POINT('Ctrl Pts',(-4.97473164011615E-6,1.17000356538632,
4.99499072157072));
#27046=CARTESIAN_POINT('Ctrl Pts',(0.0127769627408511,1.17000164210058,
4.9949925373019));
#27047=CARTESIAN_POINT('Ctrl Pts',(0.0350570588945874,1.16961980751136,
4.99716004002923));
#27048=CARTESIAN_POINT('Ctrl Pts',(0.0872618962792086,1.16729578401546,
5.01077833249387));
#27049=CARTESIAN_POINT('Ctrl Pts',(0.122360056952786,1.16381776209691,5.03300796539089));
#27050=CARTESIAN_POINT('Ctrl Pts',(0.161538770355668,1.15911150646468,5.07115681742508));
#27051=CARTESIAN_POINT('Ctrl Pts',(0.177759019988499,1.15672868520667,5.09416769688216));
#27052=CARTESIAN_POINT('Ctrl Pts',(0.199547314450672,1.1533125745775,5.14538224923639));
#27053=CARTESIAN_POINT('Ctrl Pts',(0.204999999999999,1.15235992827903,5.17355041476736));
#27054=CARTESIAN_POINT('Ctrl Pts',(0.204999999999999,1.15235992827903,5.2));
#27055=CARTESIAN_POINT('Ctrl Pts',(0.234492626320026,1.17686584120771,5.2));
#27056=CARTESIAN_POINT('Ctrl Pts',(0.234492626320026,1.17686584120771,5.17037400265145));
#27057=CARTESIAN_POINT('Ctrl Pts',(0.228592229859133,1.1780835276557,5.13881431659721));
#27058=CARTESIAN_POINT('Ctrl Pts',(0.204662083875366,1.18248576762501,5.08088946271256));
#27059=CARTESIAN_POINT('Ctrl Pts',(0.186690885906675,1.18557585757076,5.05453934674594));
#27060=CARTESIAN_POINT('Ctrl Pts',(0.142497929826391,1.19174220944178,5.01030250445097));
#27061=CARTESIAN_POINT('Ctrl Pts',(0.102259384899266,1.19636361322958,4.98396469296537));
#27062=CARTESIAN_POINT('Ctrl Pts',(0.0335828950866025,1.19987839029729,
4.96556047978417));
#27063=CARTESIAN_POINT('Ctrl Pts',(-0.0222401922789184,1.20045910805244,
4.96273883536335));
#27064=CARTESIAN_POINT('Ctrl Pts',(-0.0915400219194833,1.19713526569684,
4.97952753552852));
#27065=CARTESIAN_POINT('Ctrl Pts',(-0.152167749680949,1.19070622188097,
5.01676689334197));
#27066=CARTESIAN_POINT('Ctrl Pts',(-0.196601450552936,1.18397925051513,
5.06597720676137));
#27067=CARTESIAN_POINT('Ctrl Pts',(-0.228111094333853,1.17818452128479,
5.13119983678783));
#27068=CARTESIAN_POINT('Ctrl Pts',(-0.234294478758728,1.17688759738335,
5.17767894605582));
#27069=CARTESIAN_POINT('Ctrl Pts',(-0.234425323120645,1.17685953455129,
5.22956894464554));
#27070=CARTESIAN_POINT('Ctrl Pts',(-0.228496361591337,1.17808596546445,
5.26111603578263));
#27071=CARTESIAN_POINT('Ctrl Pts',(-0.204599918973935,1.18248717481483,
5.31905282963216));
#27072=CARTESIAN_POINT('Ctrl Pts',(-0.186607973526257,1.18557851967241,
5.34540463031795));
#27073=CARTESIAN_POINT('Ctrl Pts',(-0.145105499862307,1.19138154283581,
5.38703853259485));
#27074=CARTESIAN_POINT('Ctrl Pts',(-0.118808426842686,1.19445759764994,
5.40509087371658));
#27075=CARTESIAN_POINT('Ctrl Pts',(-0.0673004953048968,1.19832870594691,
5.42640311279717));
#27076=CARTESIAN_POINT('Ctrl Pts',(-0.0286029864222697,1.20010475087302,
5.43548184690207));
#27077=CARTESIAN_POINT('Ctrl Pts',(0.0270809220838994,1.20001767329007,
5.43500694450787));
#27078=CARTESIAN_POINT('Ctrl Pts',(0.0797919333124946,1.19779759041496,
5.42375237476982));
#27079=CARTESIAN_POINT('Ctrl Pts',(0.132977608595357,1.19291479882069,5.39638849063154));
#27080=CARTESIAN_POINT('Ctrl Pts',(0.175078618630889,1.18735985109294,5.35981780168936));
#27081=CARTESIAN_POINT('Ctrl Pts',(0.208561308949327,1.18184858998349,5.31286098873592));
#27082=CARTESIAN_POINT('Ctrl Pts',(0.230065594000457,1.17776475629821,5.25703220095455));
#27083=CARTESIAN_POINT('Ctrl Pts',(0.234492626320026,1.17686584120771,5.21851592037048));
#27084=CARTESIAN_POINT('Ctrl Pts',(0.234492626320026,1.17686584120771,5.2));
#27085=CARTESIAN_POINT('Origin',(0.,0.,5.7));
#27086=CARTESIAN_POINT('',(-1.2,1.46957615897682E-16,4.78));
#27087=CARTESIAN_POINT('Origin',(0.,0.,4.78));
#27088=CARTESIAN_POINT('',(-1.2,1.46957615897682E-16,5.7));
#27089=CARTESIAN_POINT('',(-0.770454411370329,0.92,5.67));
#27090=CARTESIAN_POINT('Origin',(0.,0.,4.75000000000001));
#27091=CARTESIAN_POINT('',(0.770454411370329,0.92,5.67));
#27092=CARTESIAN_POINT('Origin',(0.,0.,5.67));
#27093=CARTESIAN_POINT('Origin',(0.,0.,4.75000000000001));
#27094=CARTESIAN_POINT('Origin',(0.,0.95,5.2));
#27095=CARTESIAN_POINT('',(0.052199831018601,0.728126483839824,5.39824272405723));
#27096=CARTESIAN_POINT('',(4.49108658880295E-5,0.73001022386789,4.99496886927581));
#27097=CARTESIAN_POINT('Ctrl Pts',(0.052199831018601,0.728126483839824,
5.39824272405723));
#27098=CARTESIAN_POINT('Ctrl Pts',(0.0982302293711315,0.724809534278522,
5.38612233463488));
#27099=CARTESIAN_POINT('Ctrl Pts',(0.138345638847835,0.717149230706244,
5.35791819673363));
#27100=CARTESIAN_POINT('Ctrl Pts',(0.179663146502877,0.70696778967891,5.30171478600323));
#27101=CARTESIAN_POINT('Ctrl Pts',(0.190478690331408,0.703787523302871,
5.27956401023439));
#27102=CARTESIAN_POINT('Ctrl Pts',(0.200029921602327,0.700875879246346,
5.24612373179211));
#27103=CARTESIAN_POINT('Ctrl Pts',(0.202134771215936,0.700214283582941,
5.23577968142387));
#27104=CARTESIAN_POINT('Ctrl Pts',(0.207647089542785,0.698446891625313,
5.19157712891713));
#27105=CARTESIAN_POINT('Ctrl Pts',(0.203489755447152,0.699929714878053,
5.15701245250423));
#27106=CARTESIAN_POINT('Ctrl Pts',(0.180823445480298,0.70658166075718,5.09972093035022));
#27107=CARTESIAN_POINT('Ctrl Pts',(0.165889838070269,0.710634834844429,
5.07678258040992));
#27108=CARTESIAN_POINT('Ctrl Pts',(0.133222196340668,0.717699405062405,
5.04269842669383));
#27109=CARTESIAN_POINT('Ctrl Pts',(0.0959130924875414,0.724650186751937,
5.0140371229421));
#27110=CARTESIAN_POINT('Ctrl Pts',(0.0407143958653069,0.729423560490129,
4.9970978585716));
#27111=CARTESIAN_POINT('Ctrl Pts',(0.0087683139836932,0.730010101818503,
4.99497497756199));
#27112=CARTESIAN_POINT('Ctrl Pts',(4.4910865888031E-5,0.73001022386789,
4.99496886927581));
#27113=CARTESIAN_POINT('Ctrl Pts',(4.4910865888031E-5,0.73001022386789,
4.99496886927581));
#27114=CARTESIAN_POINT('Ctrl Pts',(-0.0144150329885519,0.730010426177385,
4.99495874415903));
#27115=CARTESIAN_POINT('Ctrl Pts',(-0.0519814055633027,0.728864770713442,
4.99904025375886));
#27116=CARTESIAN_POINT('Ctrl Pts',(-0.100490853947505,0.723567386179355,
5.01835059987916));
#27117=CARTESIAN_POINT('Ctrl Pts',(-0.137012137156585,0.716964400696497,
5.04626166271637));
#27118=CARTESIAN_POINT('Ctrl Pts',(-0.166997619172261,0.710467577023459,
5.07729708213043));
#27119=CARTESIAN_POINT('Ctrl Pts',(-0.207199968273801,0.699117939531869,
5.14702206281837));
#27120=CARTESIAN_POINT('Ctrl Pts',(-0.209088681335109,0.698093356717381,
5.21440963098396));
#27121=CARTESIAN_POINT('Ctrl Pts',(-0.188472856825575,0.704386618397043,
5.28674848041702));
#27122=CARTESIAN_POINT('Ctrl Pts',(-0.172527170805406,0.709084583389726,
5.31545761418984));
#27123=CARTESIAN_POINT('Ctrl Pts',(-0.126074871673654,0.719302690250943,
5.3654558850147));
#27124=CARTESIAN_POINT('Ctrl Pts',(-0.0624049065864234,0.730148572765185,
5.40608102393392));
#27125=CARTESIAN_POINT('Ctrl Pts',(0.0162020118434573,0.730720485951348,
5.40772140776134));
#27126=CARTESIAN_POINT('Ctrl Pts',(0.052199831018601,0.728126483839824,
5.39824272405723));
#27127=CARTESIAN_POINT('',(-2.51052593825206E-17,0.95,4.995));
#27128=CARTESIAN_POINT('Origin',(0.,0.,5.685));
#27129=CARTESIAN_POINT('',(-0.682934843158555,0.95,5.7));
#27130=CARTESIAN_POINT('Ctrl Pts',(-0.682934843158555,0.95,5.7));
#27131=CARTESIAN_POINT('Ctrl Pts',(-0.726694627264442,0.935903263540092,
5.68590326354009));
#27132=CARTESIAN_POINT('Ctrl Pts',(-0.770454411370329,0.92,5.67));
#27133=CARTESIAN_POINT('',(0.682934843158555,0.95,5.7));
#27134=CARTESIAN_POINT('Origin',(0.,0.,5.7));
#27135=CARTESIAN_POINT('Ctrl Pts',(0.770454411370329,0.92,5.67));
#27136=CARTESIAN_POINT('Ctrl Pts',(0.726694627264442,0.935903263540092,
5.68590326354009));
#27137=CARTESIAN_POINT('Ctrl Pts',(0.682934843158555,0.950000000000001,
5.7));
#27138=CARTESIAN_POINT('Origin',(0.,3.6089936932244E-17,4.7543933982822));
#27139=CARTESIAN_POINT('',(-1.1787867965644,0.,4.7287867965644));
#27140=CARTESIAN_POINT('Origin',(0.,7.2179873864488E-17,4.7287867965644));
#27141=CARTESIAN_POINT('',(-1.1893933982822,2.17838555677817E-16,4.7543933982822));
#27142=CARTESIAN_POINT('Origin',(0.,0.,4.725));
#27143=CARTESIAN_POINT('',(-1.1712132034356,2.86864500141304E-16,4.7212132034356));
#27144=CARTESIAN_POINT('Origin',(0.,7.1716125035326E-17,4.7212132034356));
#27145=CARTESIAN_POINT('',(-1.175,1.43895998899814E-16,4.725));
#27146=CARTESIAN_POINT('Ctrl Pts',(0.0574844932621232,0.697635673567799,
5.42785529611499));
#27147=CARTESIAN_POINT('Ctrl Pts',(0.108362285081162,0.693443393568619,
5.41500017367323));
#27148=CARTESIAN_POINT('Ctrl Pts',(0.153783173631022,0.683700872584965,
5.38492528292425));
#27149=CARTESIAN_POINT('Ctrl Pts',(0.202453501259093,0.670296320458785,
5.32107996750068));
#27150=CARTESIAN_POINT('Ctrl Pts',(0.215583701847853,0.666020452558282,
5.29529098994732));
#27151=CARTESIAN_POINT('Ctrl Pts',(0.227321703930627,0.662060184763746,
5.25551407980518));
#27152=CARTESIAN_POINT('Ctrl Pts',(0.229928314309894,0.66115513119461,5.24311976375499));
#27153=CARTESIAN_POINT('Ctrl Pts',(0.236794050807431,0.658726504222929,
5.18991348571448));
#27154=CARTESIAN_POINT('Ctrl Pts',(0.231462706037527,0.66080100427468,5.14789144672313));
#27155=CARTESIAN_POINT('Ctrl Pts',(0.203869008088291,0.669781865995222,
5.08051031045204));
#27156=CARTESIAN_POINT('Ctrl Pts',(0.18605041127256,0.675154593136393,5.05431187603876));
#27157=CARTESIAN_POINT('Ctrl Pts',(0.14822387585714,0.684346822022482,5.01626492020255));
#27158=CARTESIAN_POINT('Ctrl Pts',(0.105765749697592,0.693258892245674,
4.98506844977587));
#27159=CARTESIAN_POINT('Ctrl Pts',(0.028738398930405,0.700850964995508,
4.96254287357644));
#27160=CARTESIAN_POINT('Ctrl Pts',(-0.0475862280670742,0.699755567657756,
4.96563476101538));
#27161=CARTESIAN_POINT('Ctrl Pts',(-0.111011416912225,0.691877659824728,
4.98973284239457));
#27162=CARTESIAN_POINT('Ctrl Pts',(-0.152587648961219,0.683387533301053,
5.02024984047599));
#27163=CARTESIAN_POINT('Ctrl Pts',(-0.18727301159214,0.674952805171226,
5.054836260095));
#27164=CARTESIAN_POINT('Ctrl Pts',(-0.235690308368254,0.659782116656368,
5.13510787390001));
#27165=CARTESIAN_POINT('Ctrl Pts',(-0.238469103754452,0.658266427814801,
5.21784077794351));
#27166=CARTESIAN_POINT('Ctrl Pts',(-0.213091855455513,0.666842690298363,
5.30389851392055));
#27167=CARTESIAN_POINT('Ctrl Pts',(-0.19378027571931,0.673129747072274,
5.33701028923091));
#27168=CARTESIAN_POINT('Ctrl Pts',(-0.13987348404776,0.686445436448048,
5.39292755581025));
#27169=CARTESIAN_POINT('Ctrl Pts',(-0.0681937113019595,0.700215139205497,
5.43630057604647));
#27170=CARTESIAN_POINT('Ctrl Pts',(0.0176957967597459,0.700914223020843,
5.43790857372489));
#27171=CARTESIAN_POINT('Ctrl Pts',(0.0574844932621232,0.697635673567799,
5.42785529611499));
#27172=CARTESIAN_POINT('Ctrl Pts',(0.0557229391809491,0.707799276991807,
5.4179844387624));
#27173=CARTESIAN_POINT('Ctrl Pts',(0.105006256977315,0.703890847153119,
5.40537480552625));
#27174=CARTESIAN_POINT('Ctrl Pts',(0.148647188430249,0.694846643807852,
5.3759195474566));
#27175=CARTESIAN_POINT('Ctrl Pts',(0.194854073400739,0.682520843360022,
5.31462589198225));
#27176=CARTESIAN_POINT('Ctrl Pts',(0.207222067153112,0.678606570745627,
5.29004247566461));
#27177=CARTESIAN_POINT('Ctrl Pts',(0.218223734130959,0.674998911137377,
5.25238582952766));
#27178=CARTESIAN_POINT('Ctrl Pts',(0.220668729091904,0.674171964569765,
5.24067000158302));
#27179=CARTESIAN_POINT('Ctrl Pts',(0.227069505891163,0.671972354474063,
5.19047530531853));
#27180=CARTESIAN_POINT('Ctrl Pts',(0.222134458180962,0.673846041938921,
5.15092792931724));
#27181=CARTESIAN_POINT('Ctrl Pts',(0.196192676791318,0.682045761228669,
5.08691771703881));
#27182=CARTESIAN_POINT('Ctrl Pts',(0.179330882194175,0.686979951172563,
5.06180111704474));
#27183=CARTESIAN_POINT('Ctrl Pts',(0.143226304178282,0.695464397761381,
5.02507782820571));
#27184=CARTESIAN_POINT('Ctrl Pts',(0.102484489395487,0.703719635746295,
4.99472610142197));
#27185=CARTESIAN_POINT('Ctrl Pts',(0.027906440222761,0.710793406085462,
4.97258182217268));
#27186=CARTESIAN_POINT('Ctrl Pts',(-0.0461857534028223,0.709770528979505,
4.97563057389981));
#27187=CARTESIAN_POINT('Ctrl Pts',(-0.107504270586471,0.702440826803183,
4.99927454745295));
#27188=CARTESIAN_POINT('Ctrl Pts',(-0.147397927045243,0.694582159236071,
5.02891815925868));
#27189=CARTESIAN_POINT('Ctrl Pts',(-0.180511954268061,0.68679303751798,
5.0623245317732));
#27190=CARTESIAN_POINT('Ctrl Pts',(-0.226207394094477,0.67288956482352,
5.13907079803442));
#27191=CARTESIAN_POINT('Ctrl Pts',(-0.228599451800739,0.671585435233324,
5.21671156965555));
#27192=CARTESIAN_POINT('Ctrl Pts',(-0.204924940023387,0.679330870447946,
5.29818796269183));
#27193=CARTESIAN_POINT('Ctrl Pts',(-0.18667582898087,0.68512183856289,5.32983099864382));
#27194=CARTESIAN_POINT('Ctrl Pts',(-0.135289824847769,0.697385634364381,
5.38378497251866));
#27195=CARTESIAN_POINT('Ctrl Pts',(-0.0662562200070666,0.710198992168331,
5.42622168260221));
#27196=CARTESIAN_POINT('Ctrl Pts',(0.017198689960621,0.710837005186152,
5.42787264463697));
#27197=CARTESIAN_POINT('Ctrl Pts',(0.0557229391809491,0.707799276991807,
5.4179844387624));
#27198=CARTESIAN_POINT('Ctrl Pts',(0.053961385099775,0.717962880415815,
5.40811358140981));
#27199=CARTESIAN_POINT('Ctrl Pts',(0.101586257474979,0.714362080694022,
5.39574770278186));
#27200=CARTESIAN_POINT('Ctrl Pts',(0.143481624048608,0.706003459483357,
5.36692393220129));
#27201=CARTESIAN_POINT('Ctrl Pts',(0.187262574361231,0.694743266777672,
5.30816886152166));
#27202=CARTESIAN_POINT('Ctrl Pts',(0.198840325026149,0.691201405115526,
5.28481252451709));
#27203=CARTESIAN_POINT('Ctrl Pts',(0.209127891401994,0.687937152872715,
5.24925198206962));
#27204=CARTESIAN_POINT('Ctrl Pts',(0.211394356433926,0.687197450207785,
5.23822944359584));
#27205=CARTESIAN_POINT('Ctrl Pts',(0.217371634459052,0.685201041374179,
5.19101530931308));
#27206=CARTESIAN_POINT('Ctrl Pts',(0.212818003303718,0.686884677213813,
5.15397596991012));
#27207=CARTESIAN_POINT('Ctrl Pts',(0.18849977677727,0.694317765523733,5.09331352376346));
#27208=CARTESIAN_POINT('Ctrl Pts',(0.172609367148655,0.698809476808259,
5.06929333940394));
#27209=CARTESIAN_POINT('Ctrl Pts',(0.138219768019526,0.706581829323507,
5.03388551869067));
#27210=CARTESIAN_POINT('Ctrl Pts',(0.0991943527896464,0.714189443251316,
5.004379471296));
#27211=CARTESIAN_POINT('Ctrl Pts',(0.0270579057126555,0.720734025456457,
4.98261272409452));
#27212=CARTESIAN_POINT('Ctrl Pts',(-0.0447870233167377,0.719788394834089,
4.98562305251957));
#27213=CARTESIAN_POINT('Ctrl Pts',(-0.103998000273259,0.7130042192009,5.00880889482078));
#27214=CARTESIAN_POINT('Ctrl Pts',(-0.142201859072561,0.705769774761479,
5.03759334393367));
#27215=CARTESIAN_POINT('Ctrl Pts',(-0.173758676496339,0.698627344676705,
5.06980881045223));
#27216=CARTESIAN_POINT('Ctrl Pts',(-0.216682882547578,0.686010491364717,
5.14305913868396));
#27217=CARTESIAN_POINT('Ctrl Pts',(-0.218958333288822,0.684774349298858,
5.21553883927192));
#27218=CARTESIAN_POINT('Ctrl Pts',(-0.1966397722577,0.691898438247459,5.29245903164574));
#27219=CARTESIAN_POINT('Ctrl Pts',(-0.179631617543846,0.69709249189911,
5.32263690477693));
#27220=CARTESIAN_POINT('Ctrl Pts',(-0.130658530873645,0.708362492334609,
5.37459846830629));
#27221=CARTESIAN_POINT('Ctrl Pts',(-0.0643423978813163,0.72016471980235,
5.41615991737817));
#27222=CARTESIAN_POINT('Ctrl Pts',(0.0166991186425822,0.720797703786039,
5.41775733684927));
#27223=CARTESIAN_POINT('Ctrl Pts',(0.053961385099775,0.717962880415815,
5.40811358140981));
#27224=CARTESIAN_POINT('Ctrl Pts',(0.052199831018601,0.728126483839824,
5.39824272405723));
#27225=CARTESIAN_POINT('Ctrl Pts',(0.0982302293711315,0.724809534278522,
5.38612233463488));
#27226=CARTESIAN_POINT('Ctrl Pts',(0.138345638847835,0.717149230706244,
5.35791819673363));
#27227=CARTESIAN_POINT('Ctrl Pts',(0.179663146502877,0.70696778967891,5.30171478600323));
#27228=CARTESIAN_POINT('Ctrl Pts',(0.190478690331408,0.703787523302871,
5.27956401023439));
#27229=CARTESIAN_POINT('Ctrl Pts',(0.200029921602327,0.700875879246346,
5.24612373179211));
#27230=CARTESIAN_POINT('Ctrl Pts',(0.202134771215936,0.700214283582941,
5.23577968142387));
#27231=CARTESIAN_POINT('Ctrl Pts',(0.207647089542785,0.698446891625313,
5.19157712891713));
#27232=CARTESIAN_POINT('Ctrl Pts',(0.203489755447152,0.699929714878053,
5.15701245250423));
#27233=CARTESIAN_POINT('Ctrl Pts',(0.180823445480298,0.70658166075718,5.09972093035022));
#27234=CARTESIAN_POINT('Ctrl Pts',(0.165889838070269,0.710634834844429,
5.07678258040992));
#27235=CARTESIAN_POINT('Ctrl Pts',(0.133222196340668,0.717699405062405,
5.04269842669383));
#27236=CARTESIAN_POINT('Ctrl Pts',(0.0959130924875414,0.724650186751937,
5.0140371229421));
#27237=CARTESIAN_POINT('Ctrl Pts',(0.0262259470050115,0.730676466546411,
4.99265167269076));
#27238=CARTESIAN_POINT('Ctrl Pts',(-0.0433865486524858,0.729803356155837,
4.995618865404));
#27239=CARTESIAN_POINT('Ctrl Pts',(-0.100490853947505,0.723567386179355,
5.01835059987916));
#27240=CARTESIAN_POINT('Ctrl Pts',(-0.137012137156585,0.716964400696497,
5.04626166271637));
#27241=CARTESIAN_POINT('Ctrl Pts',(-0.166997619172261,0.710467577023459,
5.07729708213043));
#27242=CARTESIAN_POINT('Ctrl Pts',(-0.207199968273801,0.699117939531869,
5.14702206281837));
#27243=CARTESIAN_POINT('Ctrl Pts',(-0.209088681335109,0.698093356717381,
5.21440963098396));
#27244=CARTESIAN_POINT('Ctrl Pts',(-0.188472856825575,0.704386618397043,
5.28674848041702));
#27245=CARTESIAN_POINT('Ctrl Pts',(-0.172527170805406,0.709084583389726,
5.31545761418984));
#27246=CARTESIAN_POINT('Ctrl Pts',(-0.126074871673654,0.719302690250943,
5.3654558850147));
#27247=CARTESIAN_POINT('Ctrl Pts',(-0.0624049065864234,0.730148572765185,
5.40608102393392));
#27248=CARTESIAN_POINT('Ctrl Pts',(0.0162020118434573,0.730720485951348,
5.40772140776134));
#27249=CARTESIAN_POINT('Ctrl Pts',(0.052199831018601,0.728126483839824,
5.39824272405723));
#27250=CARTESIAN_POINT('',(0.0574844932621232,0.697635673567799,5.42785529611499));
#27251=CARTESIAN_POINT('',(0.0574844932621232,0.697635673567799,5.42785529611499));
#27252=CARTESIAN_POINT('',(-0.202821321852304,0.670001188175288,5.08280703661229));
#27253=CARTESIAN_POINT('Ctrl Pts',(0.0574844932621232,0.697635673567799,
5.42785529611499));
#27254=CARTESIAN_POINT('Ctrl Pts',(0.0176957967597459,0.700914223020843,
5.43790857372489));
#27255=CARTESIAN_POINT('Ctrl Pts',(-0.0681937113019595,0.700215139205497,
5.43630057604647));
#27256=CARTESIAN_POINT('Ctrl Pts',(-0.13987348404776,0.686445436448048,
5.39292755581025));
#27257=CARTESIAN_POINT('Ctrl Pts',(-0.19378027571931,0.673129747072274,
5.33701028923091));
#27258=CARTESIAN_POINT('Ctrl Pts',(-0.213091855455513,0.666842690298363,
5.30389851392055));
#27259=CARTESIAN_POINT('Ctrl Pts',(-0.238469103754452,0.658266427814801,
5.21784077794351));
#27260=CARTESIAN_POINT('Ctrl Pts',(-0.236213308908359,0.65949684697199,
5.15067913679837));
#27261=CARTESIAN_POINT('Ctrl Pts',(-0.208439846266026,0.668297710235964,
5.09269649867272));
#27262=CARTESIAN_POINT('Ctrl Pts',(-0.202821321852304,0.670001188175288,
5.08280703661229));
#27263=CARTESIAN_POINT('',(0.202776724457231,0.669982292593922,5.08288957607631));
#27264=CARTESIAN_POINT('Ctrl Pts',(-0.202821321852304,0.670001188175288,
5.08280703661229));
#27265=CARTESIAN_POINT('Ctrl Pts',(-0.195534564259789,0.672210456996427,
5.06998122907843));
#27266=CARTESIAN_POINT('Ctrl Pts',(-0.17972259321901,0.676788903208357,
5.0473073799466));
#27267=CARTESIAN_POINT('Ctrl Pts',(-0.152587648961219,0.683387533301053,
5.02024984047599));
#27268=CARTESIAN_POINT('Ctrl Pts',(-0.111011416912225,0.691877659824728,
4.98973284239457));
#27269=CARTESIAN_POINT('Ctrl Pts',(-0.0475862280670742,0.699755567657756,
4.96563476101538));
#27270=CARTESIAN_POINT('Ctrl Pts',(0.028738398930405,0.700850964995508,
4.96254287357644));
#27271=CARTESIAN_POINT('Ctrl Pts',(0.105765749697592,0.693258892245674,
4.98506844977587));
#27272=CARTESIAN_POINT('Ctrl Pts',(0.14822387585714,0.684346822022482,5.01626492020255));
#27273=CARTESIAN_POINT('Ctrl Pts',(0.179544791652671,0.67673552419273,5.04776834727921));
#27274=CARTESIAN_POINT('Ctrl Pts',(0.192309606221861,0.673146741630874,
5.06447161752956));
#27275=CARTESIAN_POINT('Ctrl Pts',(0.202776724457231,0.669982292593922,
5.0828895760763));
#27276=CARTESIAN_POINT('Ctrl Pts',(0.202776724457231,0.669982292593922,
5.0828895760763));
#27277=CARTESIAN_POINT('Ctrl Pts',(0.207628057237965,0.668515623831736,
5.09142598925544));
#27278=CARTESIAN_POINT('Ctrl Pts',(0.211985806665345,0.667140108961854,
5.10033074597365));
#27279=CARTESIAN_POINT('Ctrl Pts',(0.231462706037527,0.66080100427468,5.14789144672313));
#27280=CARTESIAN_POINT('Ctrl Pts',(0.236794050807431,0.658726504222929,
5.18991348571448));
#27281=CARTESIAN_POINT('Ctrl Pts',(0.229928314309894,0.66115513119461,5.24311976375499));
#27282=CARTESIAN_POINT('Ctrl Pts',(0.227321703930627,0.662060184763746,
5.25551407980518));
#27283=CARTESIAN_POINT('Ctrl Pts',(0.215583701847853,0.666020452558282,
5.29529098994732));
#27284=CARTESIAN_POINT('Ctrl Pts',(0.202453501259093,0.670296320458785,
5.32107996750068));
#27285=CARTESIAN_POINT('Ctrl Pts',(0.153783173631022,0.683700872584965,
5.38492528292425));
#27286=CARTESIAN_POINT('Ctrl Pts',(0.108362285081162,0.693443393568619,
5.41500017367323));
#27287=CARTESIAN_POINT('Ctrl Pts',(0.0574844932621232,0.697635673567799,
5.42785529611499));
#27288=CARTESIAN_POINT('Origin',(0.,0.,4.7));
#27289=CARTESIAN_POINT('',(-0.7,-8.57252759403147E-17,4.74));
#27290=CARTESIAN_POINT('Origin',(0.,0.,4.74));
#27291=CARTESIAN_POINT('',(-0.7,-8.57252759403147E-17,6.1));
#27292=CARTESIAN_POINT('',(-0.7,-8.57252759403147E-17,4.7));
#27293=CARTESIAN_POINT('Origin',(0.,0.,6.1));
#27294=CARTESIAN_POINT('Origin',(0.,3.5858062517663E-17,4.7106066017178));
#27295=CARTESIAN_POINT('',(-1.12,-1.37160441504504E-16,4.7));
#27296=CARTESIAN_POINT('',(-1.1456066017178,-6.85802207522518E-17,4.7106066017178));
#27297=CARTESIAN_POINT('Origin',(0.,0.,4.7));
#27298=CARTESIAN_POINT('Origin',(0.,0.,4.7));
#27299=CARTESIAN_POINT('',(-0.74,9.06238631369041E-17,4.7));
#27300=CARTESIAN_POINT('Origin',(0.,0.,4.7));
#27301=CARTESIAN_POINT('Origin',(0.,-1.3893933982822,5.7543933982822));
#27302=CARTESIAN_POINT('',(-2.8712132034356,-1.3787867965644,5.7287867965644));
#27303=CARTESIAN_POINT('',(2.8712132034356,-1.3787867965644,5.7287867965644));
#27304=CARTESIAN_POINT('',(0.,-1.3787867965644,5.7287867965644));
#27305=CARTESIAN_POINT('',(2.82,-1.4,5.78));
#27306=CARTESIAN_POINT('',(2.8712132034356,-1.3787867965644,5.7287867965644));
#27307=CARTESIAN_POINT('',(-2.82,-1.4,5.78));
#27308=CARTESIAN_POINT('',(0.,-1.4,5.78));
#27309=CARTESIAN_POINT('',(-2.82,-1.4,5.78));
#27310=CARTESIAN_POINT('Origin',(0.,-1.3893933982822,6.2456066017178));
#27311=CARTESIAN_POINT('',(-2.82,-1.4,6.22));
#27312=CARTESIAN_POINT('',(2.82,-1.4,6.22));
#27313=CARTESIAN_POINT('',(0.,-1.4,6.22));
#27314=CARTESIAN_POINT('',(2.82,-1.4,6.22));
#27315=CARTESIAN_POINT('',(-2.8712132034356,-1.3787867965644,6.2712132034356));
#27316=CARTESIAN_POINT('Origin',(2.8456066017178,-1.3893933982822,6.9375));
#27317=CARTESIAN_POINT('',(2.8712132034356,-1.3787867965644,6.9375));
#27318=CARTESIAN_POINT('',(2.82,-1.4,6.9375));
#27319=CARTESIAN_POINT('Origin',(-2.8456066017178,-1.3893933982822,6.9375));
#27320=CARTESIAN_POINT('',(-2.8712132034356,-1.3787867965644,6.9375));
#27321=CARTESIAN_POINT('',(-2.82,-1.4,6.9375));
#27322=CARTESIAN_POINT('Origin',(-2.875,-1.375,7.575));
#27323=CARTESIAN_POINT('',(-2.8787867965644,-1.3712132034356,5.7287867965644));
#27324=CARTESIAN_POINT('',(-2.8787867965644,-1.3712132034356,8.2125));
#27325=CARTESIAN_POINT('',(-2.875,-1.375,5.725));
#27326=CARTESIAN_POINT('',(-3.27916666666667,-0.970833333333332,6.12916666666666));
#27327=CARTESIAN_POINT('',(-2.0875,-2.1625,6.5125));
#27328=CARTESIAN_POINT('Origin',(0.,-1.4,6.3));
#27329=CARTESIAN_POINT('Origin',(2.885,0.4,11.985));
#27330=CARTESIAN_POINT('',(2.895,0.225,11.975));
#27331=CARTESIAN_POINT('',(2.9,0.23,11.97));
#27332=CARTESIAN_POINT('',(3.17583333333333,0.505833333333333,11.6941666666667));
#27333=CARTESIAN_POINT('',(2.9,0.95,11.97));
#27334=CARTESIAN_POINT('',(2.9,0.4,11.97));
#27335=CARTESIAN_POINT('',(2.885,0.965,11.985));
#27336=CARTESIAN_POINT('',(3.76083333333333,0.0891666666666678,11.1091666666667));
#27337=CARTESIAN_POINT('',(2.87,0.95,12.));
#27338=CARTESIAN_POINT('',(2.31333333333332,0.393333333333335,12.5566666666667));
#27339=CARTESIAN_POINT('',(2.87,0.25,12.));
#27340=CARTESIAN_POINT('',(2.87,0.4,12.));
#27341=CARTESIAN_POINT('',(2.37999999999999,0.74,12.49));
#27342=CARTESIAN_POINT('Origin',(2.885,0.215,10.425));
#27343=CARTESIAN_POINT('',(2.8912132034356,0.221213203435596,11.9712132034356));
#27344=CARTESIAN_POINT('',(2.15083333333334,-0.519166666666663,11.2308333333333));
#27345=CARTESIAN_POINT('',(2.87,0.2,11.92));
#27346=CARTESIAN_POINT('',(2.8912132034356,0.221213203435596,11.9712132034356));
#27347=CARTESIAN_POINT('',(2.87,0.2,6.4));
#27348=CARTESIAN_POINT('',(2.87,0.2,10.425));
#27349=CARTESIAN_POINT('',(2.9,0.23,6.4));
#27350=CARTESIAN_POINT('',(2.87,0.2,6.4));
#27351=CARTESIAN_POINT('',(2.9,0.23,10.425));
#27352=CARTESIAN_POINT('Origin',(0.,0.225,11.975));
#27353=CARTESIAN_POINT('',(-2.87,0.25,12.));
#27354=CARTESIAN_POINT('',(0.,0.25,12.));
#27355=CARTESIAN_POINT('',(-2.895,0.225,11.975));
#27356=CARTESIAN_POINT('',(-2.37999999999999,0.74,12.49));
#27357=CARTESIAN_POINT('',(-2.8912132034356,0.221213203435596,11.9712132034356));
#27358=CARTESIAN_POINT('',(-2.15083333333334,-0.519166666666663,11.2308333333333));
#27359=CARTESIAN_POINT('',(0.,0.221213203435596,11.9712132034356));
#27360=CARTESIAN_POINT('Origin',(0.,1.,12.));
#27361=CARTESIAN_POINT('',(-2.87,0.95,12.));
#27362=CARTESIAN_POINT('',(0.,0.95,12.));
#27363=CARTESIAN_POINT('',(-2.87,0.4,12.));
#27364=CARTESIAN_POINT('Origin',(2.8893933982822,-0.5,5.7543933982822));
#27365=CARTESIAN_POINT('',(2.8787867965644,0.971213203435596,5.7287867965644));
#27366=CARTESIAN_POINT('',(2.8787867965644,-0.5,5.7287867965644));
#27367=CARTESIAN_POINT('',(2.9,0.95,5.78));
#27368=CARTESIAN_POINT('',(3.2153138421172,0.6346861578828,6.54123495404334));
#27369=CARTESIAN_POINT('',(2.9,-0.5,5.78));
#27370=CARTESIAN_POINT('Origin',(2.875,0.975,7.275));
#27371=CARTESIAN_POINT('',(2.9,0.95,7.275));
#27372=CARTESIAN_POINT('',(2.875,0.975,5.725));
#27373=CARTESIAN_POINT('',(3.42916666666667,0.420833333333331,6.27916666666667));
#27374=CARTESIAN_POINT('',(2.8712132034356,0.978786796564403,5.7287867965644));
#27375=CARTESIAN_POINT('',(2.1375,1.7125,6.4625));
#27376=CARTESIAN_POINT('',(2.8712132034356,0.978786796564403,11.9712132034356));
#27377=CARTESIAN_POINT('',(2.8712132034356,0.978786796564403,6.4875));
#27378=CARTESIAN_POINT('',(1.61250000000001,2.2375,10.7125));
#27379=CARTESIAN_POINT('Origin',(2.875,-0.8,5.725));
#27380=CARTESIAN_POINT('',(2.1,0.199999999999996,4.95));
#27381=CARTESIAN_POINT('',(2.875,-1.375,5.725));
#27382=CARTESIAN_POINT('',(3.27916666666667,-0.970833333333332,6.12916666666666));
#27383=CARTESIAN_POINT('',(2.3,-0.8,5.15));
#27384=CARTESIAN_POINT('Origin',(2.875,-1.375,7.575));
#27385=CARTESIAN_POINT('',(2.0875,-2.1625,6.5125));
#27386=CARTESIAN_POINT('Origin',(-2.8893933982822,-0.5,5.7543933982822));
#27387=CARTESIAN_POINT('',(-2.9,-1.32,5.78));
#27388=CARTESIAN_POINT('',(-2.9,0.95,5.78));
#27389=CARTESIAN_POINT('',(-2.9,-0.5,5.78));
#27390=CARTESIAN_POINT('',(-2.8787867965644,0.971213203435596,5.7287867965644));
#27391=CARTESIAN_POINT('',(-3.2153138421172,0.6346861578828,6.54123495404334));
#27392=CARTESIAN_POINT('',(-2.8787867965644,-0.5,5.7287867965644));
#27393=CARTESIAN_POINT('',(-2.8787867965644,-1.3712132034356,5.7287867965644));
#27394=CARTESIAN_POINT('Origin',(-2.8893933982822,-1.3456066017178,8.2125));
#27395=CARTESIAN_POINT('',(-2.9,-1.32,6.27));
#27396=CARTESIAN_POINT('',(-2.97292879382193,-1.14393431686758,6.19707120617807));
#27397=CARTESIAN_POINT('',(-2.9,-1.32,8.2125));
#27398=CARTESIAN_POINT('Origin',(-2.875,0.975,7.275));
#27399=CARTESIAN_POINT('',(-2.9,0.95,11.97));
#27400=CARTESIAN_POINT('',(-2.9,0.95,7.275));
#27401=CARTESIAN_POINT('',(-2.885,0.965,11.985));
#27402=CARTESIAN_POINT('',(-3.76083333333333,0.0891666666666678,11.1091666666667));
#27403=CARTESIAN_POINT('',(-2.8712132034356,0.978786796564404,11.9712132034356));
#27404=CARTESIAN_POINT('',(-1.61250000000001,2.2375,10.7125));
#27405=CARTESIAN_POINT('',(-2.8712132034356,0.978786796564403,5.7287867965644));
#27406=CARTESIAN_POINT('',(-2.8712132034356,0.978786796564403,6.4875));
#27407=CARTESIAN_POINT('',(-2.875,0.975,5.725));
#27408=CARTESIAN_POINT('',(-2.1375,1.7125,6.4625));
#27409=CARTESIAN_POINT('',(-3.42916666666667,0.420833333333331,6.27916666666667));
#27410=CARTESIAN_POINT('Origin',(-2.9,-0.2,8.85));
#27411=CARTESIAN_POINT('',(-2.9,0.1,6.27));
#27412=CARTESIAN_POINT('',(-2.9,2.77555756156289E-17,6.27));
#27413=CARTESIAN_POINT('',(-2.9,0.23,6.4));
#27414=CARTESIAN_POINT('Origin',(-2.9,0.1,6.4));
#27415=CARTESIAN_POINT('',(-2.9,0.23,11.97));
#27416=CARTESIAN_POINT('',(-2.9,0.23,10.425));
#27417=CARTESIAN_POINT('',(-2.9,0.4,11.97));
#27418=CARTESIAN_POINT('Origin',(-2.885,2.77555756156289E-17,6.285));
#27419=CARTESIAN_POINT('',(-2.87,0.1,6.3));
#27420=CARTESIAN_POINT('',(-2.87,2.77555756156289E-17,6.3));
#27421=CARTESIAN_POINT('',(-2.87,0.1,6.3));
#27422=CARTESIAN_POINT('Origin',(-2.885,0.4,11.985));
#27423=CARTESIAN_POINT('',(-3.17583333333333,0.505833333333333,11.6941666666667));
#27424=CARTESIAN_POINT('',(-2.31333333333332,0.393333333333335,12.5566666666667));
#27425=CARTESIAN_POINT('Origin',(-2.885,0.215,10.425));
#27426=CARTESIAN_POINT('',(-2.87,0.2,6.4));
#27427=CARTESIAN_POINT('',(-2.87,0.2,6.4));
#27428=CARTESIAN_POINT('',(-2.87,0.2,11.92));
#27429=CARTESIAN_POINT('',(-2.87,0.2,10.425));
#27430=CARTESIAN_POINT('',(-2.87,0.2,11.92));
#27431=CARTESIAN_POINT('Origin',(2.1843933982822,0.210606601717798,11.35));
#27432=CARTESIAN_POINT('',(2.21,0.2,10.67));
#27433=CARTESIAN_POINT('',(2.21,0.2,11.53));
#27434=CARTESIAN_POINT('',(2.21,0.2,11.35));
#27435=CARTESIAN_POINT('',(2.1587867965644,0.221213203435596,11.5087867965644));
#27436=CARTESIAN_POINT('',(2.21,0.2,11.53));
#27437=CARTESIAN_POINT('',(2.1587867965644,0.221213203435596,10.6912132034356));
#27438=CARTESIAN_POINT('',(2.1587867965644,0.221213203435596,11.35));
#27439=CARTESIAN_POINT('',(2.1587867965644,0.221213203435596,10.6912132034356));
#27440=CARTESIAN_POINT('Origin',(1.8156066017178,0.210606601717798,11.35));
#27441=CARTESIAN_POINT('',(1.79,0.2,11.53));
#27442=CARTESIAN_POINT('',(1.79,0.2,10.67));
#27443=CARTESIAN_POINT('',(1.79,0.2,11.35));
#27444=CARTESIAN_POINT('',(1.8412132034356,0.221213203435597,10.6912132034356));
#27445=CARTESIAN_POINT('',(1.79,0.2,10.67));
#27446=CARTESIAN_POINT('',(1.8412132034356,0.221213203435597,11.5087867965644));
#27447=CARTESIAN_POINT('',(1.8412132034356,0.221213203435597,11.35));
#27448=CARTESIAN_POINT('',(1.8412132034356,0.221213203435597,11.5087867965644));
#27449=CARTESIAN_POINT('Origin',(1.,0.215,10.685));
#27450=CARTESIAN_POINT('',(2.15,0.23,10.7));
#27451=CARTESIAN_POINT('',(1.85,0.23,10.7));
#27452=CARTESIAN_POINT('',(1.,0.23,10.7));
#27453=CARTESIAN_POINT('',(1.75333333333333,0.133333333333332,10.6033333333333));
#27454=CARTESIAN_POINT('',(1.,0.2,10.67));
#27455=CARTESIAN_POINT('',(1.99,0.390000000000002,10.86));
#27456=CARTESIAN_POINT('Origin',(1.,0.215,11.515));
#27457=CARTESIAN_POINT('',(1.,0.2,11.53));
#27458=CARTESIAN_POINT('',(1.85,0.23,11.5));
#27459=CARTESIAN_POINT('',(1.88666666666666,0.266666666666665,11.4633333333333));
#27460=CARTESIAN_POINT('',(2.15,0.23,11.5));
#27461=CARTESIAN_POINT('',(1.,0.23,11.5));
#27462=CARTESIAN_POINT('',(1.85666666666667,0.523333333333335,11.2066666666667));
#27463=CARTESIAN_POINT('Origin',(2.,0.265,11.5));
#27464=CARTESIAN_POINT('',(2.,0.38,11.5));
#27465=CARTESIAN_POINT('',(2.,0.38,11.5));
#27466=CARTESIAN_POINT('',(2.23,0.15,11.5));
#27467=CARTESIAN_POINT('Origin',(2.,0.38,10.7));
#27468=CARTESIAN_POINT('',(2.,0.38,10.7));
#27469=CARTESIAN_POINT('',(2.,0.38,10.7));
#27470=CARTESIAN_POINT('',(2.,0.38,10.7));
#27471=CARTESIAN_POINT('Origin',(0.,0.2,12.));
#27472=CARTESIAN_POINT('',(0.,0.2,6.4));
#27473=CARTESIAN_POINT('',(0.,0.2,11.92));
#27474=CARTESIAN_POINT('',(1.79,0.2,7.3));
#27475=CARTESIAN_POINT('Origin',(2.,0.2,7.3));
#27476=CARTESIAN_POINT('',(1.7,0.2,9.765));
#27477=CARTESIAN_POINT('Origin',(1.7,0.2,10.));
#27478=CARTESIAN_POINT('',(-1.98,0.2,9.7));
#27479=CARTESIAN_POINT('Origin',(-0.4,0.2,9.7));
#27480=CARTESIAN_POINT('',(2.87791997799628E-17,0.2,7.065));
#27481=CARTESIAN_POINT('Origin',(0.,0.2,7.3));
#27482=CARTESIAN_POINT('Origin',(2.,0.210606601717798,7.3));
#27483=CARTESIAN_POINT('',(1.8412132034356,0.221213203435596,7.3));
#27484=CARTESIAN_POINT('',(1.8156066017178,0.210606601717798,7.3));
#27485=CARTESIAN_POINT('Origin',(2.,0.221213203435596,7.3));
#27486=CARTESIAN_POINT('Origin',(2.,0.265,7.3));
#27487=CARTESIAN_POINT('',(2.,0.38,7.3));
#27488=CARTESIAN_POINT('',(1.885,0.265,7.3));
#27489=CARTESIAN_POINT('Origin',(0.,0.215,7.3));
#27490=CARTESIAN_POINT('',(-2.51052593825207E-17,0.23,7.095));
#27491=CARTESIAN_POINT('',(2.69422295812418E-17,0.215,7.08));
#27492=CARTESIAN_POINT('Origin',(0.,0.23,7.3));
#27493=CARTESIAN_POINT('Origin',(0.,0.6,7.3));
#27494=CARTESIAN_POINT('',(2.51052593825207E-17,0.97,7.095));
#27495=CARTESIAN_POINT('',(-2.51052593825207E-17,0.6,7.095));
#27496=CARTESIAN_POINT('Origin',(0.,0.97,7.3));
#27497=CARTESIAN_POINT('Origin',(1.7,0.215,10.));
#27498=CARTESIAN_POINT('',(1.7,0.23,9.795));
#27499=CARTESIAN_POINT('',(1.7,0.215,9.78));
#27500=CARTESIAN_POINT('Origin',(1.7,0.23,10.));
#27501=CARTESIAN_POINT('Origin',(1.7,0.6,10.));
#27502=CARTESIAN_POINT('',(1.7,0.97,9.795));
#27503=CARTESIAN_POINT('',(1.7,0.6,9.795));
#27504=CARTESIAN_POINT('Origin',(1.7,0.97,10.));
#27505=CARTESIAN_POINT('Origin',(-2.885,0.1,6.4));
#27506=CARTESIAN_POINT('Origin',(-2.87,0.1,6.4));
#27507=CARTESIAN_POINT('Origin',(0.,0.210606601717798,11.9456066017178));
#27508=CARTESIAN_POINT('Origin',(2.885,0.1,6.4));
#27509=CARTESIAN_POINT('Origin',(2.87,0.1,6.4));
#27510=CARTESIAN_POINT('Origin',(2.9,0.1,6.4));
#27511=CARTESIAN_POINT('Origin',(2.9,-0.2,8.85));
#27512=CARTESIAN_POINT('Origin',(-0.4,0.210606601717798,9.7));
#27513=CARTESIAN_POINT('',(-1.9287867965644,0.221213203435596,9.7));
#27514=CARTESIAN_POINT('Origin',(-0.4,0.221213203435597,9.7));
#27515=CARTESIAN_POINT('',(-1.9543933982822,0.210606601717798,9.7));
#27516=CARTESIAN_POINT('Origin',(-0.4,0.225,9.7));
#27517=CARTESIAN_POINT('',(-1.9212132034356,0.228786796564403,9.7));
#27518=CARTESIAN_POINT('',(-1.925,0.225,9.7));
#27519=CARTESIAN_POINT('Origin',(-0.4,0.228786796564403,9.7));
#27520=CARTESIAN_POINT('Origin',(0.,0.985,7.3));
#27521=CARTESIAN_POINT('',(-2.87791997799628E-17,1.,7.065));
#27522=CARTESIAN_POINT('Origin',(0.,1.,7.3));
#27523=CARTESIAN_POINT('',(-2.69422295812418E-17,0.985,7.08));
#27524=CARTESIAN_POINT('Origin',(0.,1.,5.7));
#27525=CARTESIAN_POINT('',(-2.82,1.,5.78));
#27526=CARTESIAN_POINT('',(2.82,1.,5.78));
#27527=CARTESIAN_POINT('',(0.,1.,5.78));
#27528=CARTESIAN_POINT('',(-2.82,1.,11.92));
#27529=CARTESIAN_POINT('',(-2.82,1.,6.4875));
#27530=CARTESIAN_POINT('',(2.82,1.,11.92));
#27531=CARTESIAN_POINT('',(0.,1.,11.92));
#27532=CARTESIAN_POINT('',(2.82,1.,6.4875));
#27533=CARTESIAN_POINT('',(1.7,1.,9.765));
#27534=CARTESIAN_POINT('Origin',(1.7,1.,10.));
#27535=CARTESIAN_POINT('',(-1.98,1.,9.7));
#27536=CARTESIAN_POINT('Origin',(-0.4,1.,9.7));
#27537=CARTESIAN_POINT('Origin',(1.7,0.985,10.));
#27538=CARTESIAN_POINT('',(1.7,0.985,9.78));
#27539=CARTESIAN_POINT('Origin',(0.,0.989393398282202,11.9456066017178));
#27540=CARTESIAN_POINT('',(0.,0.978786796564404,11.9712132034356));
#27541=CARTESIAN_POINT('',(2.8712132034356,0.978786796564404,11.9712132034356));
#27542=CARTESIAN_POINT('',(-2.82,1.,11.92));
#27543=CARTESIAN_POINT('Origin',(0.,0.989393398282202,5.7543933982822));
#27544=CARTESIAN_POINT('',(2.82,1.,5.78));
#27545=CARTESIAN_POINT('',(0.,0.978786796564403,5.7287867965644));
#27546=CARTESIAN_POINT('',(-2.8712132034356,0.978786796564403,5.7287867965644));
#27547=CARTESIAN_POINT('Origin',(2.8456066017178,0.989393398282202,6.4875));
#27548=CARTESIAN_POINT('Origin',(-2.8456066017178,0.989393398282202,6.4875));
#27549=CARTESIAN_POINT('Origin',(0.,0.975,5.725));
#27550=CARTESIAN_POINT('',(0.,0.95,5.7));
#27551=CARTESIAN_POINT('',(-2.1,0.199999999999996,4.95));
#27552=CARTESIAN_POINT('Origin',(-0.4,0.254393398282202,9.7));
#27553=CARTESIAN_POINT('',(-1.9,0.28,9.7));
#27554=CARTESIAN_POINT('',(-1.9106066017178,0.254393398282202,9.7));
#27555=CARTESIAN_POINT('Origin',(-0.4,0.28,9.7));
#27556=CARTESIAN_POINT('Origin',(-0.4,1.,9.7));
#27557=CARTESIAN_POINT('',(-1.9,0.92,9.7));
#27558=CARTESIAN_POINT('Origin',(-0.4,0.92,9.7));
#27559=CARTESIAN_POINT('',(-1.9,1.,9.7));
#27560=CARTESIAN_POINT('Origin',(-0.4,0.989393398282202,9.7));
#27561=CARTESIAN_POINT('',(-1.9287867965644,0.978786796564403,9.7));
#27562=CARTESIAN_POINT('Origin',(-0.4,0.978786796564403,9.7));
#27563=CARTESIAN_POINT('',(-1.9543933982822,0.989393398282202,9.7));
#27564=CARTESIAN_POINT('Origin',(-0.4,0.975,9.7));
#27565=CARTESIAN_POINT('',(-1.9212132034356,0.971213203435596,9.7));
#27566=CARTESIAN_POINT('',(-1.925,0.975,9.7));
#27567=CARTESIAN_POINT('Origin',(-0.4,0.971213203435596,9.7));
#27568=CARTESIAN_POINT('Origin',(-0.4,0.945606601717798,9.7));
#27569=CARTESIAN_POINT('',(-1.9106066017178,0.945606601717798,9.7));
#27570=CARTESIAN_POINT('Origin',(2.23,0.15,10.7));
#27571=CARTESIAN_POINT('',(2.23,0.15,10.7));
#27572=CARTESIAN_POINT('Origin',(2.,0.265,10.7));
#27573=CARTESIAN_POINT('Origin',(0.,0.,4.72));
#27574=CARTESIAN_POINT('',(-0.72,8.81745695386094E-17,4.72));
#27575=CARTESIAN_POINT('Origin',(0.,0.,6.1));
#27576=CARTESIAN_POINT('Origin',(0.,0.,5.7));
#27577=CARTESIAN_POINT('Origin',(0.,-1.375,5.725));
#27578=CARTESIAN_POINT('',(-2.3,-0.8,5.15));
#27579=CARTESIAN_POINT('Origin',(-2.875,-0.8,5.725));
#27580=CARTESIAN_POINT('Origin',(0.,0.975,11.975));
#27581=CARTESIAN_POINT('Origin',(0.,0.2,6.3));
#27582=CARTESIAN_POINT('',(0.,0.1,6.3));
#27583=CARTESIAN_POINT('Origin',(0.,0.1,6.4));
#38589=UNCERTAINTY_MEASURE_WITH_UNIT(LENGTH_MEASURE(0.001),#38612,
'DISTANCE_ACCURACY_VALUE',
'Maximum model space distance between geometric entities at asserted c
onnectivities');
#38595=UNCERTAINTY_MEASURE_WITH_UNIT(LENGTH_MEASURE(0.001),#38612,
'DISTANCE_ACCURACY_VALUE',
'Maximum model space distance between geometric entities at asserted c
onnectivities');
#38605=(
GEOMETRIC_REPRESENTATION_CONTEXT(3)
GLOBAL_UNCERTAINTY_ASSIGNED_CONTEXT((#38589))
GLOBAL_UNIT_ASSIGNED_CONTEXT((#38612,#38614,#38615))
REPRESENTATION_CONTEXT('','3D')
);
#38611=(
GEOMETRIC_REPRESENTATION_CONTEXT(3)
GLOBAL_UNCERTAINTY_ASSIGNED_CONTEXT((#38595))
GLOBAL_UNIT_ASSIGNED_CONTEXT((#38612,#38614,#38615))
REPRESENTATION_CONTEXT('','3D')
);
#38612=(
LENGTH_UNIT()
NAMED_UNIT(*)
SI_UNIT(.CENTI.,.METRE.)
);
#38614=(
NAMED_UNIT(*)
PLANE_ANGLE_UNIT()
SI_UNIT($,.RADIAN.)
);
#38615=(
NAMED_UNIT(*)
SI_UNIT($,.STERADIAN.)
SOLID_ANGLE_UNIT()
);
#38625=SHAPE_DEFINITION_REPRESENTATION(#38640,#38676);
#38640=PRODUCT_DEFINITION_SHAPE('',$,#38692);
#38676=SHAPE_REPRESENTATION('',(#16983),#38605);
#38682=PRODUCT_DEFINITION_CONTEXT('part definition',#38729,'design');
#38692=PRODUCT_DEFINITION('2026-10-19-02-32-41-507',
'04_Fixed_L-Bracket_Kinematic_Back_Plate',#38707,#38682);
#38707=PRODUCT_DEFINITION_FORMATION('',$,#38740);
#38729=APPLICATION_CONTEXT(
'Core Data for Automotive Mechanical Design Process');
#38730=PRODUCT_CONTEXT('part definition',#38729,'mechanical');
#38740=PRODUCT('2026-10-19-02-32-41-507',
'04_Fixed_L-Bracket_Kinematic_Back_Plate',$,(#38730));
#38851=COLOUR_RGB('Dark Blue',0.08,0.2,0.34);
#38852=FILL_AREA_STYLE_COLOUR('',#38851);
#38853=FILL_AREA_STYLE('',(#38852));
#38854=SURFACE_STYLE_FILL_AREA(#38853);
#38855=SURFACE_SIDE_STYLE('',(#38854));
#38856=SURFACE_STYLE_USAGE(.BOTH.,#38855);
#38857=PRESENTATION_STYLE_ASSIGNMENT((#38856));
ENDSEC;
END-ISO-10303-21;
